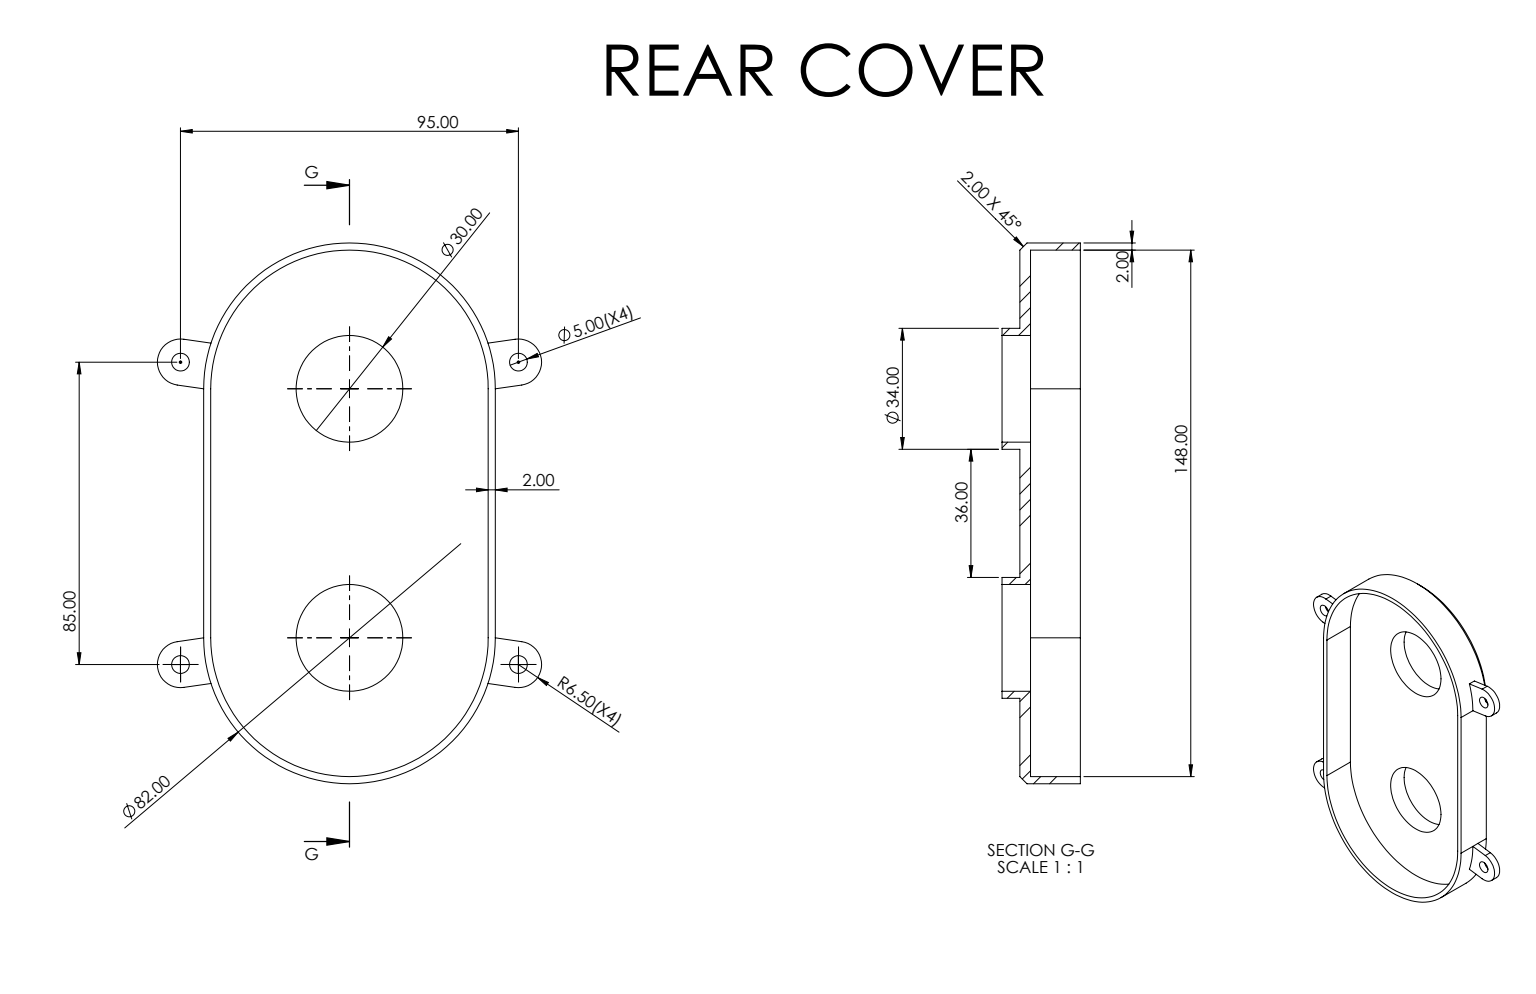
ISO-10303-21;
HEADER;
FILE_DESCRIPTION (('STEP AP214'),
    '1' );
FILE_NAME ('REAR COVER.step',
    '2026-10-24T00:51:42',
    ( '' ),
    ( '' ),
    'SwSTEP 2.0',
    'SolidWorks 2025',
    '' );
FILE_SCHEMA (( 'AUTOMOTIVE_DESIGN' ));
ENDSEC;

DATA;
#19=DIRECTION ( 'NONE',  ( -0.000000000000000000, -1.000000000000000000, -0.000000000000000000 ) ) ;
#57=VERTEX_POINT ( 'NONE', #20717 ) ;
#64=DIRECTION ( 'NONE',  ( 0.000000000000000000, 1.000000000000000000, 0.000000000000000000 ) ) ;
#78=CARTESIAN_POINT ( 'NONE',  ( 35.00000000000000000, 13.99999999999999822, 15.00000000000002132 ) ) ;
#92=EDGE_LOOP ( 'NONE', ( #21814, #17225, #4726, #11812 ) ) ;
#97=EDGE_CURVE ( 'NONE', #13097, #7488, #538, .T. ) ;
#135=EDGE_LOOP ( 'NONE', ( #20964, #9442, #3465, #7281 ) ) ;
#137=CARTESIAN_POINT ( 'NONE',  ( 42.50000000000000000, 10.00000000000000000, 47.49999999999999289 ) ) ;
#138=DIRECTION ( 'NONE',  ( -0.000000000000000000, -1.000000000000000000, -0.000000000000000000 ) ) ;
#146=VECTOR ( 'NONE', #10611, 1000.000000000000000 ) ;
#147=CARTESIAN_POINT ( 'NONE',  ( 42.50000000000000000, 7.000000000000000000, 47.49999999999999289 ) ) ;
#169=AXIS2_PLACEMENT_3D ( 'NONE', #17860, #14739, #16123 ) ;
#179=AXIS2_PLACEMENT_3D ( 'NONE', #12084, #11739, #22064 ) ;
#183=CARTESIAN_POINT ( 'NONE',  ( -42.49999999999996447, 7.000000000000000000, -47.50000000000000711 ) ) ;
#184=CYLINDRICAL_SURFACE ( 'NONE', #1331, 6.499999999999999112 ) ;
#185=AXIS2_PLACEMENT_3D ( 'NONE', #17657, #15929, #17553 ) ;
#197=LINE ( 'NONE', #10969, #5945 ) ;
#198=DIRECTION ( 'NONE',  ( -0.1421319796954322312, 0.000000000000000000, -0.9898477157360405787 ) ) ;
#202=CARTESIAN_POINT ( 'NONE',  ( -35.00000000000000000, 14.00000000000000000, 39.00000000000002132 ) ) ;
#242=EDGE_LOOP ( 'NONE', ( #11934, #16526 ) ) ;
#246=ORIENTED_EDGE ( 'NONE', *, *, #18367, .T. ) ;
#255=CARTESIAN_POINT ( 'NONE',  ( 35.00000000000000000, 17.00000000000000000, -40.99999999999997868 ) ) ;
#267=EDGE_LOOP ( 'NONE', ( #12609, #14006, #18826, #6601, #2906, #9922, #5735, #20678 ) ) ;
#279=ORIENTED_EDGE ( 'NONE', *, *, #15136, .F. ) ;
#287=AXIS2_PLACEMENT_3D ( 'NONE', #18901, #20854, #8577 ) ;
#292=DIRECTION ( 'NONE',  ( 0.000000000000000000, -1.000000000000000000, 0.000000000000000000 ) ) ;
#328=CARTESIAN_POINT ( 'NONE',  ( -35.00000000000000000, 17.00000000000000000, 2.365113165210053967E-14 ) ) ;
#336=VECTOR ( 'NONE', #1062, 1000.000000000000000 ) ;
#359=EDGE_CURVE ( 'NONE', #22631, #14416, #10776, .T. ) ;
#360=ORIENTED_EDGE ( 'NONE', *, *, #18003, .F. ) ;
#362=CARTESIAN_POINT ( 'NONE',  ( 35.00000000000000000, 0.000000000000000000, 2.365113165210053967E-14 ) ) ;
#398=EDGE_LOOP ( 'NONE', ( #11515, #3826 ) ) ;
#405=CARTESIAN_POINT ( 'NONE',  ( -41.39271818392636959, 10.00000000000000000, -5.943569790512535533 ) ) ;
#416=CYLINDRICAL_SURFACE ( 'NONE', #20007, 2.500000000000002220 ) ;
#419=ORIENTED_EDGE ( 'NONE', *, *, #14863, .F. ) ;
#424=DIRECTION ( 'NONE',  ( 0.000000000000000000, -1.000000000000000000, 0.000000000000000000 ) ) ;
#428=DIRECTION ( 'NONE',  ( 0.000000000000000000, 0.000000000000000000, -1.000000000000000000 ) ) ;
#452=DIRECTION ( 'NONE',  ( -0.000000000000000000, -1.000000000000000000, -0.000000000000000000 ) ) ;
#468=DIRECTION ( 'NONE',  ( 0.000000000000000000, 1.000000000000000000, 0.000000000000000000 ) ) ;
#472=ORIENTED_EDGE ( 'NONE', *, *, #15222, .T. ) ;
#482=ORIENTED_EDGE ( 'NONE', *, *, #4999, .F. ) ;
#484=DIRECTION ( 'NONE',  ( -0.9898477157360406897, 0.000000000000000000, -0.1421319796954317316 ) ) ;
#493=CARTESIAN_POINT ( 'NONE',  ( 47.83731665821558465, 6.999999999999999112, 38.93845529828710283 ) ) ;
#510=DIRECTION ( 'NONE',  ( 0.000000000000000000, 0.000000000000000000, 1.000000000000000000 ) ) ;
#538=CIRCLE ( 'NONE', #12595, 15.00000000000000000 ) ;
#552=FACE_BOUND ( 'NONE', #22629, .T. ) ;
#565=ADVANCED_FACE ( 'NONE', ( #8537 ), #7046, .F. ) ;
#574=CARTESIAN_POINT ( 'NONE',  ( 35.00000000000000000, 22.00000000000000355, 17.00000000000002487 ) ) ;
#594=EDGE_CURVE ( 'NONE', #9609, #19656, #19896, .T. ) ;
#608=AXIS2_PLACEMENT_3D ( 'NONE', #8171, #20770, #9889 ) ;
#628=ORIENTED_EDGE ( 'NONE', *, *, #16506, .F. ) ;
#630=DIRECTION ( 'NONE',  ( 0.000000000000000000, -1.000000000000000000, 0.000000000000000000 ) ) ;
#639=CARTESIAN_POINT ( 'NONE',  ( 42.50000000000000000, 7.000000000000000000, 49.99999999999999289 ) ) ;
#661=FACE_OUTER_BOUND ( 'NONE', #1127, .T. ) ;
#668=VERTEX_POINT ( 'NONE', #2002 ) ;
#693=CARTESIAN_POINT ( 'NONE',  ( 35.00000000000000000, 15.00000000000000000, -40.99999999999997868 ) ) ;
#716=CIRCLE ( 'NONE', #14971, 15.00000000000000000 ) ;
#718=SHAPE_REPRESENTATION_RELATIONSHIP ( 'NONE' , 'NONE' ,  #15726, #21138 ) ;
#727=FACE_OUTER_BOUND ( 'NONE', #1242, .T. ) ;
#748=EDGE_CURVE ( 'NONE', #17126, #21624, #7387, .T. ) ;
#751=FACE_OUTER_BOUND ( 'NONE', #92, .T. ) ;
#752=CARTESIAN_POINT ( 'NONE',  ( -35.00000000000000000, 17.00000000000000000, 41.00000000000002132 ) ) ;
#807=ADVANCED_FACE ( 'NONE', ( #13643, #2280 ), #20659, .T. ) ;
#809=EDGE_LOOP ( 'NONE', ( #12173, #12291, #2991, #3318 ) ) ;
#816=LINE ( 'NONE', #2658, #1235 ) ;
#837=CARTESIAN_POINT ( 'NONE',  ( -42.49999999999996447, 10.00000000000000000, -54.00000000000000711 ) ) ;
#855=ADVANCED_FACE ( 'NONE', ( #10324, #6796 ), #5093, .F. ) ;
#865=DIRECTION ( 'NONE',  ( -0.000000000000000000, 1.000000000000000000, -0.000000000000000000 ) ) ;
#883=CARTESIAN_POINT ( 'NONE',  ( -35.00000000000000000, 17.00000000000000000, -40.99999999999997868 ) ) ;
#886=FACE_OUTER_BOUND ( 'NONE', #3171, .T. ) ;
#940=DIRECTION ( 'NONE',  ( 0.000000000000000000, 0.000000000000000000, -1.000000000000000000 ) ) ;
#948=DIRECTION ( 'NONE',  ( 0.000000000000000000, 0.000000000000000000, -1.000000000000000000 ) ) ;
#963=CIRCLE ( 'NONE', #18169, 2.500000000000002220 ) ;
#968=VERTEX_POINT ( 'NONE', #6113 ) ;
#972=ORIENTED_EDGE ( 'NONE', *, *, #12220, .F. ) ;
#984=DIRECTION ( 'NONE',  ( 0.000000000000000000, 0.000000000000000000, -1.000000000000000000 ) ) ;
#1006=CIRCLE ( 'NONE', #13433, 39.00000000000000000 ) ;
#1009=CARTESIAN_POINT ( 'NONE',  ( 42.49999999999998579, 7.000000000000000000, -49.99999999999997868 ) ) ;
#1013=ORIENTED_EDGE ( 'NONE', *, *, #6207, .T. ) ;
#1017=DIRECTION ( 'NONE',  ( -0.000000000000000000, 1.000000000000000000, -0.000000000000000000 ) ) ;
#1032=CARTESIAN_POINT ( 'NONE',  ( 35.00000000000000000, 0.000000000000000000, -40.99999999999997868 ) ) ;
#1038=DIRECTION ( 'NONE',  ( 0.000000000000000000, 0.000000000000000000, -1.000000000000000000 ) ) ;
#1054=VERTEX_POINT ( 'NONE', #20767 ) ;
#1062=DIRECTION ( 'NONE',  ( -0.000000000000000000, -1.000000000000000000, -0.000000000000000000 ) ) ;
#1091=CARTESIAN_POINT ( 'NONE',  ( -28.52469787935782364, 7.000000000000000000, 4.095854054471899985 ) ) ;
#1096=DIRECTION ( 'NONE',  ( 0.000000000000000000, 0.000000000000000000, -1.000000000000000000 ) ) ;
#1120=FACE_OUTER_BOUND ( 'NONE', #7332, .T. ) ;
#1127=EDGE_LOOP ( 'NONE', ( #10984, #4974, #21316, #12105 ) ) ;
#1167=LINE ( 'NONE', #8160, #14153 ) ;
#1191=DIRECTION ( 'NONE',  ( -0.1421319796954317316, 0.000000000000000000, -0.9898477157360405787 ) ) ;
#1221=CARTESIAN_POINT ( 'NONE',  ( 41.39271818392636959, 7.000000000000000000, -5.943569790512535533 ) ) ;
#1235=VECTOR ( 'NONE', #4378, 1000.000000000000000 ) ;
#1242=EDGE_LOOP ( 'NONE', ( #6996, #21007, #22630, #22192 ) ) ;
#1265=ORIENTED_EDGE ( 'NONE', *, *, #20237, .T. ) ;
#1278=CARTESIAN_POINT ( 'NONE',  ( -35.00000000000000000, 17.00000000000000000, 41.00000000000002132 ) ) ;
#1283=VECTOR ( 'NONE', #11816, 1000.000000000000000 ) ;
#1317=DIRECTION ( 'NONE',  ( -1.000000000000000000, 0.000000000000000000, 0.000000000000000000 ) ) ;
#1331=AXIS2_PLACEMENT_3D ( 'NONE', #5809, #12782, #5471 ) ;
#1359=FACE_OUTER_BOUND ( 'NONE', #5225, .T. ) ;
#1386=CIRCLE ( 'NONE', #14175, 17.00000000000000000 ) ;
#1411=FACE_OUTER_BOUND ( 'NONE', #8286, .T. ) ;
#1430=ORIENTED_EDGE ( 'NONE', *, *, #18003, .T. ) ;
#1432=CARTESIAN_POINT ( 'NONE',  ( 35.00000000000000000, 14.00000000000000000, -38.99999999999997868 ) ) ;
#1457=ORIENTED_EDGE ( 'NONE', *, *, #7090, .T. ) ;
#1460=CARTESIAN_POINT ( 'NONE',  ( -28.52469787935786982, 10.00000000000000000, -4.095854054471906203 ) ) ;
#1464=ORIENTED_EDGE ( 'NONE', *, *, #5972, .F. ) ;
#1470=LINE ( 'NONE', #13928, #19264 ) ;
#1486=ORIENTED_EDGE ( 'NONE', *, *, #22195, .T. ) ;
#1488=( NAMED_UNIT ( * ) PLANE_ANGLE_UNIT ( ) SI_UNIT ( $, .RADIAN. ) );
#1495=DIRECTION ( 'NONE',  ( 0.000000000000000000, 0.000000000000000000, -1.000000000000000000 ) ) ;
#1522=EDGE_LOOP ( 'NONE', ( #3610, #7248, #14036, #10775 ) ) ;
#1530=ORIENTED_EDGE ( 'NONE', *, *, #20547, .F. ) ;
#1558=DIRECTION ( 'NONE',  ( 0.9898477157360406897, 0.000000000000000000, -0.1421319796954317316 ) ) ;
#1565=DIRECTION ( 'NONE',  ( 0.000000000000000000, -1.000000000000000000, 0.000000000000000000 ) ) ;
#1567=DIRECTION ( 'NONE',  ( -0.1421319796954317316, 0.000000000000000000, 0.9898477157360405787 ) ) ;
#1575=CARTESIAN_POINT ( 'NONE',  ( -35.00000000000000000, 17.00000000000000000, 2.365113165210053967E-14 ) ) ;
#1579=VECTOR ( 'NONE', #452, 1000.000000000000000 ) ;
#1582=ORIENTED_EDGE ( 'NONE', *, *, #6936, .F. ) ;
#1607=ADVANCED_FACE ( 'NONE', ( #10937 ), #2474, .F. ) ;
#1632=ADVANCED_FACE ( 'NONE', ( #751 ), #21373, .F. ) ;
#1641=CARTESIAN_POINT ( 'NONE',  ( 0.000000000000000000, 7.000000000000000000, 0.000000000000000000 ) ) ;
#1648=CARTESIAN_POINT ( 'NONE',  ( 0.000000000000000000, 0.000000000000000000, 0.000000000000000000 ) ) ;
#1691=VERTEX_POINT ( 'NONE', #17698 ) ;
#1693=CIRCLE ( 'NONE', #13357, 41.00000000000000000 ) ;
#1698=DIRECTION ( 'NONE',  ( 0.000000000000000000, 0.000000000000000000, -1.000000000000000000 ) ) ;
#1727=PRODUCT_CONTEXT ( 'NONE', #18977, 'mechanical' ) ;
#1744=LINE ( 'NONE', #12270, #4214 ) ;
#1755=DIRECTION ( 'NONE',  ( 0.1421319796954317316, 0.000000000000000000, 0.9898477157360405787 ) ) ;
#1810=EDGE_CURVE ( 'NONE', #10947, #5838, #8753, .T. ) ;
#1814=DIRECTION ( 'NONE',  ( 0.000000000000000000, -0.000000000000000000, 1.000000000000000000 ) ) ;
#1821=CARTESIAN_POINT ( 'NONE',  ( 42.49999999999998579, 10.00000000000000000, -53.99999999999997868 ) ) ;
#1844=CARTESIAN_POINT ( 'NONE',  ( -35.00000000000000000, -15.00000000000000000, 15.00000000000002132 ) ) ;
#1861=CYLINDRICAL_SURFACE ( 'NONE', #185, 17.00000000000000000 ) ;
#1869=VERTEX_POINT ( 'NONE', #4975 ) ;
#1882=ORIENTED_EDGE ( 'NONE', *, *, #8202, .F. ) ;
#1921=VECTOR ( 'NONE', #2869, 1000.000000000000000 ) ;
#1930=CARTESIAN_POINT ( 'NONE',  ( -35.00000000000000000, 14.00000000000000000, 2.365113165210053967E-14 ) ) ;
#1932=DIRECTION ( 'NONE',  ( 0.000000000000000000, 1.000000000000000000, 0.000000000000000000 ) ) ;
#1934=CARTESIAN_POINT ( 'NONE',  ( 41.39271818392636959, 10.00000000000000000, -5.943569790512535533 ) ) ;
#1937=AXIS2_PLACEMENT_3D ( 'NONE', #10361, #1558, #17361 ) ;
#1949=CARTESIAN_POINT ( 'NONE',  ( 35.00000000000000000, -15.00000000000000000, 2.255140518769849223E-14 ) ) ;
#1979=DIRECTION ( 'NONE',  ( 0.000000000000000000, 0.000000000000000000, 1.000000000000000000 ) ) ;
#1986=LINE ( 'NONE', #16071, #20757 ) ;
#1989=VECTOR ( 'NONE', #13933, 1000.000000000000000 ) ;
#2002=CARTESIAN_POINT ( 'NONE',  ( 36.06598984771572702, 7.000000000000000000, -48.42385786802028491 ) ) ;
#2042=DIRECTION ( 'NONE',  ( 0.000000000000000000, -0.000000000000000000, -1.000000000000000000 ) ) ;
#2066=DIRECTION ( 'NONE',  ( 1.000000000000000000, 0.000000000000000000, 0.000000000000000000 ) ) ;
#2069=CARTESIAN_POINT ( 'NONE',  ( -47.83731665821558465, 10.00000000000000000, 38.93845529828710283 ) ) ;
#2070=ADVANCED_FACE ( 'NONE', ( #4157, #11129 ), #5758, .T. ) ;
#2076=CARTESIAN_POINT ( 'NONE',  ( 42.50000000000000000, 10.00000000000000000, 44.99999999999999289 ) ) ;
#2124=DIRECTION ( 'NONE',  ( -0.1421319796954322312, 0.000000000000000000, 0.9898477157360405787 ) ) ;
#2151=ORIENTED_EDGE ( 'NONE', *, *, #14754, .T. ) ;
#2156=CARTESIAN_POINT ( 'NONE',  ( -35.00000000000000000, 0.000000000000000000, -40.99999999999997868 ) ) ;
#2157=CARTESIAN_POINT ( 'NONE',  ( 0.000000000000000000, 10.00000000000000000, 0.000000000000000000 ) ) ;
#2214=FACE_OUTER_BOUND ( 'NONE', #13033, .T. ) ;
#2237=CARTESIAN_POINT ( 'NONE',  ( -35.00000000000000000, 13.99999999999999822, 2.255140518769849223E-14 ) ) ;
#2242=CARTESIAN_POINT ( 'NONE',  ( 42.49999999999998579, 10.00000000000000000, -53.99999999999997868 ) ) ;
#2247=CARTESIAN_POINT ( 'NONE',  ( -42.49999999999996447, 10.00000000000000000, -47.50000000000000711 ) ) ;
#2268=DIRECTION ( 'NONE',  ( 0.000000000000000000, -1.000000000000000000, 0.000000000000000000 ) ) ;
#2271=CARTESIAN_POINT ( 'NONE',  ( 42.50000000000000000, 7.000000000000000000, 47.49999999999999289 ) ) ;
#2272=DIRECTION ( 'NONE',  ( 0.000000000000000000, 0.000000000000000000, 1.000000000000000000 ) ) ;
#2280=FACE_BOUND ( 'NONE', #20023, .T. ) ;
#2309=VECTOR ( 'NONE', #22199, 1000.000000000000000 ) ;
#2314=CIRCLE ( 'NONE', #18793, 39.00000000000001421 ) ;
#2320=ORIENTED_EDGE ( 'NONE', *, *, #16902, .T. ) ;
#2333=DIRECTION ( 'NONE',  ( -0.000000000000000000, 1.000000000000000000, -0.000000000000000000 ) ) ;
#2334=CARTESIAN_POINT ( 'NONE',  ( -35.00000000000000000, -15.00000000000000000, 2.255140518769849223E-14 ) ) ;
#2351=CARTESIAN_POINT ( 'NONE',  ( 41.39271818392635538, 10.00000000000000000, 5.943569790512533757 ) ) ;
#2360=ORIENTED_EDGE ( 'NONE', *, *, #12885, .T. ) ;
#2367=VECTOR ( 'NONE', #10808, 1000.000000000000000 ) ;
#2431=AXIS2_PLACEMENT_3D ( 'NONE', #11425, #7878, #7759 ) ;
#2470=EDGE_CURVE ( 'NONE', #5472, #3556, #22295, .T. ) ;
#2471=EDGE_LOOP ( 'NONE', ( #2738, #11209 ) ) ;
#2474=CYLINDRICAL_SURFACE ( 'NONE', #16918, 15.00000000000000000 ) ;
#2482=VECTOR ( 'NONE', #1567, 1000.000000000000114 ) ;
#2485=AXIS2_PLACEMENT_3D ( 'NONE', #6864, #20850, #13709 ) ;
#2513=CARTESIAN_POINT ( 'NONE',  ( -35.00000000000000000, 22.00000000000000711, 2.255140518769849223E-14 ) ) ;
#2520=LINE ( 'NONE', #4463, #14838 ) ;
#2557=DIRECTION ( 'NONE',  ( 0.000000000000000000, -1.000000000000000000, 0.000000000000000000 ) ) ;
#2637=EDGE_CURVE ( 'NONE', #16920, #5292, #18981, .T. ) ;
#2651=DIRECTION ( 'NONE',  ( 0.000000000000000000, -1.000000000000000000, 0.000000000000000000 ) ) ;
#2653=EDGE_CURVE ( 'NONE', #14416, #22631, #5060, .T. ) ;
#2658=CARTESIAN_POINT ( 'NONE',  ( -36.06598984771573413, 10.00000000000000000, 48.42385786802029912 ) ) ;
#2734=CARTESIAN_POINT ( 'NONE',  ( 35.00000000000000000, 13.99999999999999822, -14.99999999999997691 ) ) ;
#2737=DIRECTION ( 'NONE',  ( 0.000000000000000000, 1.000000000000000000, 0.000000000000000000 ) ) ;
#2738=ORIENTED_EDGE ( 'NONE', *, *, #7323, .F. ) ;
#2767=ORIENTED_EDGE ( 'NONE', *, *, #22107, .F. ) ;
#2795=DIRECTION ( 'NONE',  ( -0.000000000000000000, 1.000000000000000000, -0.000000000000000000 ) ) ;
#2798=VECTOR ( 'NONE', #7146, 1000.000000000000000 ) ;
#2800=PRODUCT_DEFINITION_CONTEXT ( 'detailed design', #13389, 'design' ) ;
#2815=ORIENTED_EDGE ( 'NONE', *, *, #3808, .F. ) ;
#2833=LINE ( 'NONE', #13339, #2309 ) ;
#2869=DIRECTION ( 'NONE',  ( -0.000000000000000000, -1.000000000000000000, -0.000000000000000000 ) ) ;
#2879=ADVANCED_FACE ( 'NONE', ( #22518 ), #19072, .F. ) ;
#2888=VECTOR ( 'NONE', #11317, 1000.000000000000000 ) ;
#2890=AXIS2_PLACEMENT_3D ( 'NONE', #7003, #6777, #13959 ) ;
#2892=EDGE_LOOP ( 'NONE', ( #1882, #5395 ) ) ;
#2899=EDGE_CURVE ( 'NONE', #1869, #7355, #7256, .T. ) ;
#2906=ORIENTED_EDGE ( 'NONE', *, *, #3732, .T. ) ;
#2956=PLANE ( 'NONE',  #21445 ) ;
#2991=ORIENTED_EDGE ( 'NONE', *, *, #3871, .T. ) ;
#3007=ORIENTED_EDGE ( 'NONE', *, *, #12807, .F. ) ;
#3018=ORIENTED_EDGE ( 'NONE', *, *, #5005, .F. ) ;
#3027=EDGE_LOOP ( 'NONE', ( #19847, #19122, #3846, #7657 ) ) ;
#3041=FACE_BOUND ( 'NONE', #7156, .T. ) ;
#3052=ORIENTED_EDGE ( 'NONE', *, *, #5972, .T. ) ;
#3065=CARTESIAN_POINT ( 'NONE',  ( -42.50000000000000000, 10.00000000000000000, 47.49999999999999289 ) ) ;
#3069=CARTESIAN_POINT ( 'NONE',  ( -42.50000000000000000, 10.00000000000000000, 47.49999999999999289 ) ) ;
#3072=AXIS2_PLACEMENT_3D ( 'NONE', #4866, #20225, #18842 ) ;
#3079=FACE_OUTER_BOUND ( 'NONE', #16197, .T. ) ;
#3083=ORIENTED_EDGE ( 'NONE', *, *, #12925, .F. ) ;
#3092=EDGE_LOOP ( 'NONE', ( #20794, #13463 ) ) ;
#3117=ORIENTED_EDGE ( 'NONE', *, *, #14660, .F. ) ;
#3130=DIRECTION ( 'NONE',  ( 0.9898477157360406897, 0.000000000000000000, 0.1421319796954317316 ) ) ;
#3134=EDGE_CURVE ( 'NONE', #9062, #12985, #18351, .T. ) ;
#3151=VERTEX_POINT ( 'NONE', #22144 ) ;
#3162=EDGE_CURVE ( 'NONE', #6209, #12263, #7939, .T. ) ;
#3168=VECTOR ( 'NONE', #14054, 999.9999999999998863 ) ;
#3171=EDGE_LOOP ( 'NONE', ( #3117, #19504, #7395, #8158 ) ) ;
#3185=DIRECTION ( 'NONE',  ( 0.000000000000000000, 1.000000000000000000, 0.000000000000000000 ) ) ;
#3196=EDGE_LOOP ( 'NONE', ( #19684, #11491, #11820, #18594 ) ) ;
#3240=EDGE_CURVE ( 'NONE', #5472, #968, #3575, .T. ) ;
#3258=EDGE_LOOP ( 'NONE', ( #279, #7361, #12926, #9656 ) ) ;
#3270=LINE ( 'NONE', #12405, #4800 ) ;
#3305=FACE_OUTER_BOUND ( 'NONE', #5612, .T. ) ;
#3310=PLANE ( 'NONE',  #8420 ) ;
#3318=ORIENTED_EDGE ( 'NONE', *, *, #5798, .T. ) ;
#3325=EDGE_LOOP ( 'NONE', ( #14607, #3483, #8538, #18494, #14886 ) ) ;
#3380=CARTESIAN_POINT ( 'NONE',  ( 42.49999999999998579, 10.00000000000000000, -47.49999999999997868 ) ) ;
#3382=ORIENTED_EDGE ( 'NONE', *, *, #8745, .F. ) ;
#3420=ORIENTED_EDGE ( 'NONE', *, *, #22107, .T. ) ;
#3455=CIRCLE ( 'NONE', #8931, 41.00000000000000000 ) ;
#3465=ORIENTED_EDGE ( 'NONE', *, *, #4547, .T. ) ;
#3482=ADVANCED_FACE ( 'NONE', ( #10754 ), #19600, .T. ) ;
#3483=ORIENTED_EDGE ( 'NONE', *, *, #3782, .F. ) ;
#3492=EDGE_CURVE ( 'NONE', #8659, #11088, #9060, .T. ) ;
#3507=CARTESIAN_POINT ( 'NONE',  ( 42.49999999999998579, 10.00000000000000000, -44.99999999999997868 ) ) ;
#3509=DIRECTION ( 'NONE',  ( 0.000000000000000000, 0.000000000000000000, -1.000000000000000000 ) ) ;
#3529=CARTESIAN_POINT ( 'NONE',  ( -42.50000000000000000, 10.00000000000000000, 47.49999999999999289 ) ) ;
#3535=CIRCLE ( 'NONE', #6816, 17.00000000000000000 ) ;
#3551=CYLINDRICAL_SURFACE ( 'NONE', #287, 6.499999999999999112 ) ;
#3554=DIRECTION ( 'NONE',  ( 0.1421319796954317316, 0.000000000000000000, -0.9898477157360405787 ) ) ;
#3556=VERTEX_POINT ( 'NONE', #574 ) ;
#3575=LINE ( 'NONE', #8602, #7278 ) ;
#3598=VECTOR ( 'NONE', #7421, 1000.000000000000000 ) ;
#3610=ORIENTED_EDGE ( 'NONE', *, *, #97, .T. ) ;
#3623=EDGE_CURVE ( 'NONE', #22687, #9796, #7787, .T. ) ;
#3625=FACE_BOUND ( 'NONE', #8762, .T. ) ;
#3626=DIRECTION ( 'NONE',  ( 0.000000000000000000, -1.000000000000000000, 0.000000000000000000 ) ) ;
#3632=ORIENTED_EDGE ( 'NONE', *, *, #16597, .F. ) ;
#3633=ORIENTED_EDGE ( 'NONE', *, *, #2637, .T. ) ;
#3653=CARTESIAN_POINT ( 'NONE',  ( -42.49999999999996447, 10.00000000000000000, -50.00000000000000711 ) ) ;
#3654=DIRECTION ( 'NONE',  ( 0.000000000000000000, 0.000000000000000000, -1.000000000000000000 ) ) ;
#3666=CARTESIAN_POINT ( 'NONE',  ( 35.00000000000000000, 17.00000000000000000, -38.99999999999999289 ) ) ;
#3694=CARTESIAN_POINT ( 'NONE',  ( -41.39271818392631985, 7.000000000000000000, 5.943569790512528428 ) ) ;
#3701=ORIENTED_EDGE ( 'NONE', *, *, #14762, .T. ) ;
#3723=DIRECTION ( 'NONE',  ( 0.000000000000000000, 0.000000000000000000, -1.000000000000000000 ) ) ;
#3732=EDGE_CURVE ( 'NONE', #8574, #9457, #11569, .T. ) ;
#3744=LINE ( 'NONE', #9429, #22652 ) ;
#3754=CARTESIAN_POINT ( 'NONE',  ( -42.49999999999996447, 7.000000000000000000, -47.50000000000000711 ) ) ;
#3772=ORIENTED_EDGE ( 'NONE', *, *, #9384, .T. ) ;
#3782=EDGE_CURVE ( 'NONE', #9695, #9796, #15672, .T. ) ;
#3797=CIRCLE ( 'NONE', #16596, 2.500000000000002220 ) ;
#3808=EDGE_CURVE ( 'NONE', #8847, #16743, #12022, .T. ) ;
#3812=MECHANICAL_DESIGN_GEOMETRIC_PRESENTATION_REPRESENTATION('',(#13668),#11862);
#3826=ORIENTED_EDGE ( 'NONE', *, *, #4433, .F. ) ;
#3832=EDGE_LOOP ( 'NONE', ( #10837, #10650, #12585, #7543 ) ) ;
#3833=CARTESIAN_POINT ( 'NONE',  ( 35.00000000000000000, 0.000000000000000000, 2.365113165210053967E-14 ) ) ;
#3846=ORIENTED_EDGE ( 'NONE', *, *, #3162, .T. ) ;
#3858=LINE ( 'NONE', #11145, #15632 ) ;
#3871=EDGE_CURVE ( 'NONE', #1691, #6084, #197, .T. ) ;
#3877=AXIS2_PLACEMENT_3D ( 'NONE', #5239, #3185, #19221 ) ;
#3904=AXIS2_PLACEMENT_3D ( 'NONE', #2334, #21939, #12752 ) ;
#3908=CYLINDRICAL_SURFACE ( 'NONE', #3989, 15.00000000000000000 ) ;
#3909=VERTEX_POINT ( 'NONE', #7192 ) ;
#3938=ORIENTED_EDGE ( 'NONE', *, *, #15815, .F. ) ;
#3948=VECTOR ( 'NONE', #21942, 1000.000000000000000 ) ;
#3967=VERTEX_POINT ( 'NONE', #19463 ) ;
#3985=CIRCLE ( 'NONE', #5431, 41.00000000000000000 ) ;
#3989=AXIS2_PLACEMENT_3D ( 'NONE', #1949, #7334, #5502 ) ;
#3991=VERTEX_POINT ( 'NONE', #13233 ) ;
#4001=PLANE ( 'NONE',  #6171 ) ;
#4010=ADVANCED_FACE ( 'NONE', ( #661 ), #13131, .F. ) ;
#4031=FACE_OUTER_BOUND ( 'NONE', #1522, .T. ) ;
#4051=ORIENTED_EDGE ( 'NONE', *, *, #20533, .F. ) ;
#4074=VECTOR ( 'NONE', #2557, 1000.000000000000000 ) ;
#4101=CARTESIAN_POINT ( 'NONE',  ( -35.00000000000000000, 25.00000000000000000, 2.365113165210053967E-14 ) ) ;
#4114=DIRECTION ( 'NONE',  ( 0.000000000000000000, 0.000000000000000000, -1.000000000000000000 ) ) ;
#4116=FACE_OUTER_BOUND ( 'NONE', #19797, .T. ) ;
#4157=FACE_BOUND ( 'NONE', #9390, .T. ) ;
#4173=FACE_OUTER_BOUND ( 'NONE', #135, .T. ) ;
#4176=CARTESIAN_POINT ( 'NONE',  ( -35.00000000000000000, 10.00000000000000000, -40.99999999999997868 ) ) ;
#4180=CIRCLE ( 'NONE', #10015, 17.00000000000000000 ) ;
#4196=DIRECTION ( 'NONE',  ( 0.9898477157360405787, 0.000000000000000000, 0.1421319796954322312 ) ) ;
#4214=VECTOR ( 'NONE', #19, 1000.000000000000000 ) ;
#4228=DIRECTION ( 'NONE',  ( -0.000000000000000000, -1.000000000000000000, -0.000000000000000000 ) ) ;
#4246=CARTESIAN_POINT ( 'NONE',  ( 48.93401015228424455, 10.00000000000000000, -46.57614213197967956 ) ) ;
#4273=EDGE_CURVE ( 'NONE', #10917, #1054, #3858, .T. ) ;
#4280=CARTESIAN_POINT ( 'NONE',  ( -41.39271818392636959, 10.00000000000000000, -5.943569790512535533 ) ) ;
#4289=CARTESIAN_POINT ( 'NONE',  ( -35.00000000000000000, 15.00000000000000000, 2.365113165210053967E-14 ) ) ;
#4293=CIRCLE ( 'NONE', #4608, 6.499999999999999112 ) ;
#4294=ORIENTED_EDGE ( 'NONE', *, *, #6266, .F. ) ;
#4295=CYLINDRICAL_SURFACE ( 'NONE', #11531, 2.500000000000002220 ) ;
#4300=VECTOR ( 'NONE', #18816, 1000.000000000000000 ) ;
#4320=FACE_OUTER_BOUND ( 'NONE', #18037, .T. ) ;
#4355=LINE ( 'NONE', #9843, #5362 ) ;
#4356=EDGE_CURVE ( 'NONE', #8405, #10917, #16739, .T. ) ;
#4359=ORIENTED_EDGE ( 'NONE', *, *, #9254, .F. ) ;
#4378=DIRECTION ( 'NONE',  ( 0.000000000000000000, -1.000000000000000000, 0.000000000000000000 ) ) ;
#4381=VERTEX_POINT ( 'NONE', #9191 ) ;
#4406=ORIENTED_EDGE ( 'NONE', *, *, #9942, .T. ) ;
#4409=DIRECTION ( 'NONE',  ( 0.000000000000000000, 0.000000000000000000, -1.000000000000000000 ) ) ;
#4418=ORIENTED_EDGE ( 'NONE', *, *, #3492, .T. ) ;
#4426=EDGE_CURVE ( 'NONE', #8747, #14227, #18943, .T. ) ;
#4433=EDGE_CURVE ( 'NONE', #11772, #6084, #7969, .T. ) ;
#4438=ORIENTED_EDGE ( 'NONE', *, *, #17655, .F. ) ;
#4453=VECTOR ( 'NONE', #10143, 1000.000000000000114 ) ;
#4463=CARTESIAN_POINT ( 'NONE',  ( -35.00000000000000000, 0.000000000000000000, -40.99999999999997868 ) ) ;
#4491=( LENGTH_UNIT ( ) NAMED_UNIT ( * ) SI_UNIT ( .MILLI., .METRE. ) );
#4495=VECTOR ( 'NONE', #8025, 1000.000000000000000 ) ;
#4510=ORIENTED_EDGE ( 'NONE', *, *, #22195, .F. ) ;
#4526=ORIENTED_EDGE ( 'NONE', *, *, #2470, .F. ) ;
#4529=ORIENTED_EDGE ( 'NONE', *, *, #9755, .F. ) ;
#4547=EDGE_CURVE ( 'NONE', #13043, #9609, #8486, .T. ) ;
#4554=ORIENTED_EDGE ( 'NONE', *, *, #5776, .T. ) ;
#4582=CYLINDRICAL_SURFACE ( 'NONE', #4905, 41.00000000000000000 ) ;
#4598=DIRECTION ( 'NONE',  ( -0.000000000000000000, 1.000000000000000000, -0.000000000000000000 ) ) ;
#4604=AXIS2_PLACEMENT_3D ( 'NONE', #11825, #4963, #18944 ) ;
#4608=AXIS2_PLACEMENT_3D ( 'NONE', #147, #7142, #7375 ) ;
#4630=CARTESIAN_POINT ( 'NONE',  ( 48.93401015228426587, 7.000000000000000000, 46.57614213197968667 ) ) ;
#4638=PLANE ( 'NONE',  #21326 ) ;
#4644=AXIS2_PLACEMENT_3D ( 'NONE', #5773, #2333, #14584 ) ;
#4650=DIRECTION ( 'NONE',  ( 0.000000000000000000, 1.000000000000000000, 0.000000000000000000 ) ) ;
#4653=PLANE ( 'NONE',  #6608 ) ;
#4675=CARTESIAN_POINT ( 'NONE',  ( -35.00000000000000000, 15.00000000000000000, -40.99999999999997868 ) ) ;
#4687=AXIS2_PLACEMENT_3D ( 'NONE', #18782, #10056, #5042 ) ;
#4695=EDGE_LOOP ( 'NONE', ( #17693, #20869, #7283, #1582 ) ) ;
#4697=DIRECTION ( 'NONE',  ( 0.000000000000000000, 0.000000000000000000, -1.000000000000000000 ) ) ;
#4711=EDGE_CURVE ( 'NONE', #8574, #668, #9822, .T. ) ;
#4716=CARTESIAN_POINT ( 'NONE',  ( 35.00000000000000000, -15.00000000000000000, 2.255140518769849223E-14 ) ) ;
#4726=ORIENTED_EDGE ( 'NONE', *, *, #13705, .F. ) ;
#4743=DIRECTION ( 'NONE',  ( 0.000000000000000000, 1.000000000000000000, 0.000000000000000000 ) ) ;
#4749=CARTESIAN_POINT ( 'NONE',  ( 42.49999999999998579, 10.00000000000000000, -49.99999999999997868 ) ) ;
#4750=CARTESIAN_POINT ( 'NONE',  ( 35.00000000000000000, 15.00000000000000000, 41.00000000000002132 ) ) ;
#4756=EDGE_LOOP ( 'NONE', ( #6381, #1486, #17696, #9217 ) ) ;
#4776=EDGE_CURVE ( 'NONE', #5656, #13337, #18797, .T. ) ;
#4800=VECTOR ( 'NONE', #19302, 999.9999999999998863 ) ;
#4837=VERTEX_POINT ( 'NONE', #2242 ) ;
#4841=ADVANCED_FACE ( 'NONE', ( #12651 ), #7514, .F. ) ;
#4843=LINE ( 'NONE', #11813, #4300 ) ;
#4846=CARTESIAN_POINT ( 'NONE',  ( -35.00000000000000000, -15.00000000000000000, -14.99999999999997691 ) ) ;
#4854=PLANE ( 'NONE',  #10166 ) ;
#4863=CARTESIAN_POINT ( 'NONE',  ( 35.00000000000000000, 7.000000000000000000, 41.00000000000002132 ) ) ;
#4866=CARTESIAN_POINT ( 'NONE',  ( 35.00000000000000000, 17.00000000000000000, 2.365113165210053967E-14 ) ) ;
#4869=CARTESIAN_POINT ( 'NONE',  ( -35.00000000000000000, 22.00000000000000355, 2.365113165210053967E-14 ) ) ;
#4897=CYLINDRICAL_SURFACE ( 'NONE', #12016, 2.500000000000002220 ) ;
#4905=AXIS2_PLACEMENT_3D ( 'NONE', #10050, #13370, #4697 ) ;
#4906=DIRECTION ( 'NONE',  ( 0.000000000000000000, 0.000000000000000000, -1.000000000000000000 ) ) ;
#4961=CARTESIAN_POINT ( 'NONE',  ( -35.00000000000000000, 0.000000000000000000, 2.365113165210053967E-14 ) ) ;
#4963=DIRECTION ( 'NONE',  ( 0.000000000000000000, -1.000000000000000000, 0.000000000000000000 ) ) ;
#4973=CARTESIAN_POINT ( 'NONE',  ( 48.93401015228424455, 10.00000000000000000, -46.57614213197967956 ) ) ;
#4974=ORIENTED_EDGE ( 'NONE', *, *, #17616, .F. ) ;
#4975=CARTESIAN_POINT ( 'NONE',  ( 35.00000000000001421, 0.000000000000000000, 39.00000000000002132 ) ) ;
#4995=DIRECTION ( 'NONE',  ( 0.000000000000000000, -0.000000000000000000, -1.000000000000000000 ) ) ;
#4999=EDGE_CURVE ( 'NONE', #12985, #6209, #9557, .T. ) ;
#5005=EDGE_CURVE ( 'NONE', #57, #13636, #3270, .T. ) ;
#5024=VERTEX_POINT ( 'NONE', #10570 ) ;
#5042=DIRECTION ( 'NONE',  ( 0.000000000000000000, 0.000000000000000000, -1.000000000000000000 ) ) ;
#5060=CIRCLE ( 'NONE', #22275, 2.500000000000002220 ) ;
#5088=AXIS2_PLACEMENT_3D ( 'NONE', #21868, #6167, #3723 ) ;
#5093=PLANE ( 'NONE',  #12578 ) ;
#5096=ORIENTED_EDGE ( 'NONE', *, *, #12555, .F. ) ;
#5129=DIRECTION ( 'NONE',  ( 0.000000000000000000, 0.000000000000000000, 1.000000000000000000 ) ) ;
#5132=FACE_OUTER_BOUND ( 'NONE', #12353, .T. ) ;
#5153=VECTOR ( 'NONE', #16231, 1000.000000000000114 ) ;
#5154=CARTESIAN_POINT ( 'NONE',  ( 35.00000000000000000, 17.00000000000000000, -38.99999999999999289 ) ) ;
#5160=PLANE ( 'NONE',  #16283 ) ;
#5166=ORIENTED_EDGE ( 'NONE', *, *, #5233, .T. ) ;
#5176=DIRECTION ( 'NONE',  ( 0.000000000000000000, 0.000000000000000000, -1.000000000000000000 ) ) ;
#5191=ORIENTED_EDGE ( 'NONE', *, *, #10332, .T. ) ;
#5223=ADVANCED_FACE ( 'NONE', ( #727 ), #5529, .T. ) ;
#5225=EDGE_LOOP ( 'NONE', ( #419, #21595, #15652, #18243 ) ) ;
#5233=EDGE_CURVE ( 'NONE', #15126, #668, #21690, .T. ) ;
#5239=CARTESIAN_POINT ( 'NONE',  ( -35.00000000000000000, 17.00000000000000000, 2.365113165210053967E-14 ) ) ;
#5245=ADVANCED_FACE ( 'NONE', ( #2214 ), #9196, .T. ) ;
#5292=VERTEX_POINT ( 'NONE', #7940 ) ;
#5312=DIRECTION ( 'NONE',  ( -1.000000000000000000, -0.000000000000000000, -0.000000000000000000 ) ) ;
#5318=CARTESIAN_POINT ( 'NONE',  ( -35.00000000000000000, 10.00000000000000000, 2.365113165210053967E-14 ) ) ;
#5323=CARTESIAN_POINT ( 'NONE',  ( -35.00000000000000000, 7.000000000000000000, 2.365113165210053967E-14 ) ) ;
#5329=DIRECTION ( 'NONE',  ( 1.000000000000000000, -0.000000000000000000, -0.000000000000000000 ) ) ;
#5354=DIRECTION ( 'NONE',  ( 0.000000000000000000, -1.000000000000000000, 0.000000000000000000 ) ) ;
#5362=VECTOR ( 'NONE', #13243, 1000.000000000000000 ) ;
#5368=FACE_OUTER_BOUND ( 'NONE', #19665, .T. ) ;
#5372=LINE ( 'NONE', #3666, #8701 ) ;
#5379=EDGE_CURVE ( 'NONE', #13337, #21700, #1167, .T. ) ;
#5395=ORIENTED_EDGE ( 'NONE', *, *, #7223, .F. ) ;
#5403=ORIENTED_EDGE ( 'NONE', *, *, #10283, .T. ) ;
#5406=PLANE ( 'NONE',  #13322 ) ;
#5410=AXIS2_PLACEMENT_3D ( 'NONE', #10783, #5636, #1979 ) ;
#5431=AXIS2_PLACEMENT_3D ( 'NONE', #5323, #8763, #15735 ) ;
#5436=CARTESIAN_POINT ( 'NONE',  ( 35.00000000000000000, 17.00000000000000000, 2.365113165210053967E-14 ) ) ;
#5471=DIRECTION ( 'NONE',  ( 0.000000000000000000, 0.000000000000000000, -1.000000000000000000 ) ) ;
#5472=VERTEX_POINT ( 'NONE', #15582 ) ;
#5502=DIRECTION ( 'NONE',  ( 0.000000000000000000, 0.000000000000000000, 1.000000000000000000 ) ) ;
#5529=CYLINDRICAL_SURFACE ( 'NONE', #9801, 6.499999999999999112 ) ;
#5536=ORIENTED_EDGE ( 'NONE', *, *, #3492, .F. ) ;
#5581=CARTESIAN_POINT ( 'NONE',  ( -35.00000000000000000, 6.999999999999999112, 41.00000000000002132 ) ) ;
#5582=DIRECTION ( 'NONE',  ( 0.000000000000000000, -1.000000000000000000, 0.000000000000000000 ) ) ;
#5596=AXIS2_PLACEMENT_3D ( 'NONE', #362, #7353, #14321 ) ;
#5597=EDGE_CURVE ( 'NONE', #22687, #4837, #14537, .T. ) ;
#5602=AXIS2_PLACEMENT_3D ( 'NONE', #405, #4196, #12990 ) ;
#5603=EDGE_LOOP ( 'NONE', ( #2360, #9910, #6653, #18837 ) ) ;
#5612=EDGE_LOOP ( 'NONE', ( #4406, #14116, #16090, #19294 ) ) ;
#5623=AXIS2_PLACEMENT_3D ( 'NONE', #12093, #12312, #10248 ) ;
#5636=DIRECTION ( 'NONE',  ( 0.000000000000000000, -1.000000000000000000, 0.000000000000000000 ) ) ;
#5643=DIRECTION ( 'NONE',  ( 0.000000000000000000, 0.000000000000000000, -1.000000000000000000 ) ) ;
#5656=VERTEX_POINT ( 'NONE', #18676 ) ;
#5666=ORIENTED_EDGE ( 'NONE', *, *, #3240, .T. ) ;
#5687=EDGE_CURVE ( 'NONE', #21104, #668, #8339, .T. ) ;
#5735=ORIENTED_EDGE ( 'NONE', *, *, #5379, .F. ) ;
#5749=CARTESIAN_POINT ( 'NONE',  ( 42.50000000000000000, 10.00000000000000000, 47.49999999999999289 ) ) ;
#5758=PLANE ( 'NONE',  #21652 ) ;
#5773=CARTESIAN_POINT ( 'NONE',  ( -42.49999999999996447, 7.000000000000000000, -47.50000000000000711 ) ) ;
#5776=EDGE_CURVE ( 'NONE', #10413, #20463, #6888, .T. ) ;
#5781=CIRCLE ( 'NONE', #21513, 6.499999999999999112 ) ;
#5798=EDGE_CURVE ( 'NONE', #6084, #11772, #6509, .T. ) ;
#5809=CARTESIAN_POINT ( 'NONE',  ( 42.50000000000000000, 10.00000000000000000, 47.49999999999999289 ) ) ;
#5820=ADVANCED_FACE ( 'NONE', ( #13939 ), #3551, .T. ) ;
#5834=DIRECTION ( 'NONE',  ( 0.000000000000000000, -1.000000000000000000, 0.000000000000000000 ) ) ;
#5838=VERTEX_POINT ( 'NONE', #13714 ) ;
#5849=VERTEX_POINT ( 'NONE', #6869 ) ;
#5877=DIRECTION ( 'NONE',  ( 0.000000000000000000, -1.000000000000000000, 0.000000000000000000 ) ) ;
#5899=ORIENTED_EDGE ( 'NONE', *, *, #17210, .T. ) ;
#5910=CARTESIAN_POINT ( 'NONE',  ( -35.00000000000000000, 7.000000000000000000, 2.365113165210053967E-14 ) ) ;
#5918=DIRECTION ( 'NONE',  ( -0.000000000000000000, 1.000000000000000000, -0.000000000000000000 ) ) ;
#5924=ADVANCED_FACE ( 'NONE', ( #12348 ), #4001, .T. ) ;
#5945=VECTOR ( 'NONE', #5582, 1000.000000000000000 ) ;
#5963=EDGE_CURVE ( 'NONE', #16920, #6360, #18189, .T. ) ;
#5972=EDGE_CURVE ( 'NONE', #3909, #16743, #21985, .T. ) ;
#5988=DIRECTION ( 'NONE',  ( 0.000000000000000000, -1.000000000000000000, 0.000000000000000000 ) ) ;
#5993=ORIENTED_EDGE ( 'NONE', *, *, #2653, .F. ) ;
#5996=DIRECTION ( 'NONE',  ( 0.000000000000000000, 0.000000000000000000, 1.000000000000000000 ) ) ;
#6003=CIRCLE ( 'NONE', #19531, 17.00000000000000000 ) ;
#6013=ORIENTED_EDGE ( 'NONE', *, *, #16529, .F. ) ;
#6016=DIRECTION ( 'NONE',  ( 0.000000000000000000, 0.000000000000000000, -1.000000000000000000 ) ) ;
#6054=DIRECTION ( 'NONE',  ( 0.000000000000000000, 0.000000000000000000, 1.000000000000000000 ) ) ;
#6057=ORIENTED_EDGE ( 'NONE', *, *, #9831, .T. ) ;
#6076=ADVANCED_FACE ( 'NONE', ( #1120 ), #18966, .F. ) ;
#6080=ORIENTED_EDGE ( 'NONE', *, *, #8804, .F. ) ;
#6084=VERTEX_POINT ( 'NONE', #11967 ) ;
#6085=CARTESIAN_POINT ( 'NONE',  ( 42.49999999999998579, 7.000000000000000000, -47.49999999999997868 ) ) ;
#6088=CARTESIAN_POINT ( 'NONE',  ( -48.93401015228422324, 7.000000000000000000, -46.57614213197970088 ) ) ;
#6093=VECTOR ( 'NONE', #9580, 1000.000000000000000 ) ;
#6107=ADVANCED_FACE ( 'NONE', ( #886 ), #7879, .T. ) ;
#6113=CARTESIAN_POINT ( 'NONE',  ( 35.00000000000000000, 17.00000000000000000, -16.99999999999997868 ) ) ;
#6123=DIRECTION ( 'NONE',  ( -0.9898477157360406897, 0.000000000000000000, 0.1421319796954317316 ) ) ;
#6156=ORIENTED_EDGE ( 'NONE', *, *, #7339, .F. ) ;
#6167=DIRECTION ( 'NONE',  ( -0.000000000000000000, -1.000000000000000000, -0.000000000000000000 ) ) ;
#6171=AXIS2_PLACEMENT_3D ( 'NONE', #14392, #16354, #198 ) ;
#6180=DIRECTION ( 'NONE',  ( -1.000000000000000000, -0.000000000000000000, -0.000000000000000000 ) ) ;
#6181=VECTOR ( 'NONE', #1565, 1000.000000000000000 ) ;
#6183=ORIENTED_EDGE ( 'NONE', *, *, #15884, .T. ) ;
#6207=EDGE_CURVE ( 'NONE', #8659, #3991, #3985, .T. ) ;
#6209=VERTEX_POINT ( 'NONE', #13994 ) ;
#6223=CARTESIAN_POINT ( 'NONE',  ( -35.00000000000000000, 17.00000000000000000, 39.00000000000003553 ) ) ;
#6240=EDGE_CURVE ( 'NONE', #15452, #17708, #21350, .T. ) ;
#6253=CARTESIAN_POINT ( 'NONE',  ( 35.00000000000000000, 10.00000000000000000, -40.99999999999997868 ) ) ;
#6254=ORIENTED_EDGE ( 'NONE', *, *, #8021, .F. ) ;
#6264=ORIENTED_EDGE ( 'NONE', *, *, #21917, .T. ) ;
#6266=EDGE_CURVE ( 'NONE', #9062, #16838, #14181, .T. ) ;
#6267=ORIENTED_EDGE ( 'NONE', *, *, #12925, .T. ) ;
#6293=EDGE_LOOP ( 'NONE', ( #10660, #3420 ) ) ;
#6298=DIRECTION ( 'NONE',  ( -1.067522139062650671E-15, 0.000000000000000000, -1.000000000000000000 ) ) ;
#6360=VERTEX_POINT ( 'NONE', #11493 ) ;
#6381=ORIENTED_EDGE ( 'NONE', *, *, #15884, .F. ) ;
#6432=VECTOR ( 'NONE', #6881, 1000.000000000000000 ) ;
#6485=ORIENTED_EDGE ( 'NONE', *, *, #15815, .T. ) ;
#6494=CARTESIAN_POINT ( 'NONE',  ( 28.52469787935785561, 7.000000000000000000, 4.095854054471903538 ) ) ;
#6498=DIRECTION ( 'NONE',  ( 0.000000000000000000, -1.000000000000000000, 0.000000000000000000 ) ) ;
#6503=ORIENTED_EDGE ( 'NONE', *, *, #20630, .T. ) ;
#6509=CIRCLE ( 'NONE', #4687, 2.500000000000002220 ) ;
#6512=CARTESIAN_POINT ( 'NONE',  ( 47.83731665821556334, 10.00000000000000000, -38.93845529828706020 ) ) ;
#6514=DIRECTION ( 'NONE',  ( 0.000000000000000000, 0.000000000000000000, -1.000000000000000000 ) ) ;
#6548=ORIENTED_EDGE ( 'NONE', *, *, #14606, .F. ) ;
#6549=ADVANCED_FACE ( 'NONE', ( #3079 ), #4582, .T. ) ;
#6573=VERTEX_POINT ( 'NONE', #16937 ) ;
#6576=DIRECTION ( 'NONE',  ( -0.000000000000000000, -1.000000000000000000, -0.000000000000000000 ) ) ;
#6592=ORIENTED_EDGE ( 'NONE', *, *, #6645, .F. ) ;
#6597=EDGE_CURVE ( 'NONE', #4837, #21104, #12122, .T. ) ;
#6599=ORIENTED_EDGE ( 'NONE', *, *, #8202, .T. ) ;
#6601=ORIENTED_EDGE ( 'NONE', *, *, #8021, .T. ) ;
#6608=AXIS2_PLACEMENT_3D ( 'NONE', #18848, #20121, #14510 ) ;
#6609=CARTESIAN_POINT ( 'NONE',  ( 35.00000000000000000, 10.00000000000000000, 41.00000000000002132 ) ) ;
#6611=CARTESIAN_POINT ( 'NONE',  ( 28.52469787935786982, 7.000000000000000000, -4.095854054471906203 ) ) ;
#6619=LINE ( 'NONE', #12332, #14910 ) ;
#6645=EDGE_CURVE ( 'NONE', #21941, #21842, #14040, .T. ) ;
#6653=ORIENTED_EDGE ( 'NONE', *, *, #19285, .F. ) ;
#6655=ORIENTED_EDGE ( 'NONE', *, *, #18444, .T. ) ;
#6662=LINE ( 'NONE', #9974, #13839 ) ;
#6690=ORIENTED_EDGE ( 'NONE', *, *, #20419, .T. ) ;
#6706=FACE_OUTER_BOUND ( 'NONE', #13210, .T. ) ;
#6711=ORIENTED_EDGE ( 'NONE', *, *, #12855, .F. ) ;
#6725=FACE_BOUND ( 'NONE', #8721, .T. ) ;
#6743=AXIS2_PLACEMENT_3D ( 'NONE', #1641, #10865, #12066 ) ;
#6751=CARTESIAN_POINT ( 'NONE',  ( 42.50000000000000000, 10.00000000000000000, 47.49999999999999289 ) ) ;
#6760=CARTESIAN_POINT ( 'NONE',  ( -36.06598984771573413, 10.00000000000000000, 48.42385786802029912 ) ) ;
#6777=DIRECTION ( 'NONE',  ( 0.000000000000000000, -1.000000000000000000, 0.000000000000000000 ) ) ;
#6796=FACE_OUTER_BOUND ( 'NONE', #8539, .T. ) ;
#6802=ORIENTED_EDGE ( 'NONE', *, *, #6240, .F. ) ;
#6805=ADVANCED_FACE ( 'NONE', ( #19799 ), #14725, .T. ) ;
#6816=AXIS2_PLACEMENT_3D ( 'NONE', #5436, #19196, #10463 ) ;
#6829=AXIS2_PLACEMENT_3D ( 'NONE', #15245, #4743, #11711 ) ;
#6836=ORIENTED_EDGE ( 'NONE', *, *, #97, .F. ) ;
#6845=FACE_OUTER_BOUND ( 'NONE', #7681, .T. ) ;
#6858=CARTESIAN_POINT ( 'NONE',  ( -35.00000000000000000, 13.99999999999999822, 15.00000000000002132 ) ) ;
#6864=CARTESIAN_POINT ( 'NONE',  ( 42.49999999999998579, 10.00000000000000000, -47.49999999999997868 ) ) ;
#6867=AXIS2_PLACEMENT_3D ( 'NONE', #13399, #22025, #22256 ) ;
#6869=CARTESIAN_POINT ( 'NONE',  ( -42.49999999999996447, 7.000000000000000000, -45.00000000000000711 ) ) ;
#6871=DIRECTION ( 'NONE',  ( 0.000000000000000000, -0.000000000000000000, -1.000000000000000000 ) ) ;
#6881=DIRECTION ( 'NONE',  ( 0.000000000000000000, -1.000000000000000000, 0.000000000000000000 ) ) ;
#6885=ORIENTED_EDGE ( 'NONE', *, *, #17210, .F. ) ;
#6888=CIRCLE ( 'NONE', #9447, 2.500000000000002220 ) ;
#6906=CARTESIAN_POINT ( 'NONE',  ( 41.39271818392635538, 10.00000000000000000, 5.943569790512533757 ) ) ;
#6923=CONICAL_SURFACE ( 'NONE', #19372, 39.00000000000001421, 0.7853981633974447263 ) ;
#6936=EDGE_CURVE ( 'NONE', #21565, #6573, #2833, .T. ) ;
#6974=ORIENTED_EDGE ( 'NONE', *, *, #12885, .F. ) ;
#6981=DIRECTION ( 'NONE',  ( 0.000000000000000000, -0.000000000000000000, -1.000000000000000000 ) ) ;
#6991=VERTEX_POINT ( 'NONE', #11865 ) ;
#6996=ORIENTED_EDGE ( 'NONE', *, *, #21917, .F. ) ;
#7003=CARTESIAN_POINT ( 'NONE',  ( 0.000000000000000000, 7.000000000000000000, 0.000000000000000000 ) ) ;
#7046=CYLINDRICAL_SURFACE ( 'NONE', #20278, 2.500000000000002220 ) ;
#7056=ADVANCED_FACE ( 'NONE', ( #21040 ), #21149, .F. ) ;
#7061=DIRECTION ( 'NONE',  ( 0.000000000000000000, 0.000000000000000000, -1.000000000000000000 ) ) ;
#7066=FACE_OUTER_BOUND ( 'NONE', #14925, .T. ) ;
#7085=PRODUCT_DEFINITION_SHAPE ( 'NONE', 'NONE',  #12887 ) ;
#7090=EDGE_CURVE ( 'NONE', #1691, #19883, #20599, .T. ) ;
#7104=CARTESIAN_POINT ( 'NONE',  ( 35.00000000000000000, -15.00000000000000000, 15.00000000000002132 ) ) ;
#7132=DIRECTION ( 'NONE',  ( 0.000000000000000000, -1.000000000000000000, 0.000000000000000000 ) ) ;
#7142=DIRECTION ( 'NONE',  ( 0.000000000000000000, -1.000000000000000000, 0.000000000000000000 ) ) ;
#7146=DIRECTION ( 'NONE',  ( -0.000000000000000000, -1.000000000000000000, -0.000000000000000000 ) ) ;
#7151=CIRCLE ( 'NONE', #3877, 17.00000000000000000 ) ;
#7156=EDGE_LOOP ( 'NONE', ( #1457, #12012 ) ) ;
#7158=VECTOR ( 'NONE', #12878, 1000.000000000000000 ) ;
#7167=AXIS2_PLACEMENT_3D ( 'NONE', #16932, #10045, #20494 ) ;
#7183=ADVANCED_FACE ( 'NONE', ( #16092 ), #7285, .F. ) ;
#7192=CARTESIAN_POINT ( 'NONE',  ( -35.00000000000000711, 0.000000000000000000, -38.99999999999997868 ) ) ;
#7195=FACE_BOUND ( 'NONE', #14076, .T. ) ;
#7197=ADVANCED_FACE ( 'NONE', ( #9567 ), #11049, .F. ) ;
#7203=ORIENTED_EDGE ( 'NONE', *, *, #16597, .T. ) ;
#7223=EDGE_CURVE ( 'NONE', #8088, #13043, #22084, .T. ) ;
#7248=ORIENTED_EDGE ( 'NONE', *, *, #13670, .T. ) ;
#7256=LINE ( 'NONE', #18012, #13820 ) ;
#7278=VECTOR ( 'NONE', #17303, 1000.000000000000000 ) ;
#7281=ORIENTED_EDGE ( 'NONE', *, *, #594, .T. ) ;
#7283=ORIENTED_EDGE ( 'NONE', *, *, #18365, .T. ) ;
#7285=PLANE ( 'NONE',  #16206 ) ;
#7288=DIRECTION ( 'NONE',  ( 0.000000000000000000, 0.000000000000000000, -1.000000000000000000 ) ) ;
#7301=EDGE_CURVE ( 'NONE', #6991, #968, #7802, .T. ) ;
#7314=CARTESIAN_POINT ( 'NONE',  ( -35.00000000000000000, 0.000000000000000000, 41.00000000000002132 ) ) ;
#7319=DIRECTION ( 'NONE',  ( 0.000000000000000000, 0.000000000000000000, -1.000000000000000000 ) ) ;
#7323=EDGE_CURVE ( 'NONE', #6360, #3151, #6003, .T. ) ;
#7332=EDGE_LOOP ( 'NONE', ( #9773, #8300, #5096, #18585 ) ) ;
#7334=DIRECTION ( 'NONE',  ( -0.000000000000000000, 1.000000000000000000, -0.000000000000000000 ) ) ;
#7339=EDGE_CURVE ( 'NONE', #13337, #21842, #16893, .T. ) ;
#7353=DIRECTION ( 'NONE',  ( 0.000000000000000000, -1.000000000000000000, 0.000000000000000000 ) ) ;
#7355=VERTEX_POINT ( 'NONE', #10115 ) ;
#7358=EDGE_CURVE ( 'NONE', #20463, #10413, #19172, .T. ) ;
#7361=ORIENTED_EDGE ( 'NONE', *, *, #13952, .T. ) ;
#7375=DIRECTION ( 'NONE',  ( 0.000000000000000000, 0.000000000000000000, -1.000000000000000000 ) ) ;
#7387=LINE ( 'NONE', #9214, #2367 ) ;
#7395=ORIENTED_EDGE ( 'NONE', *, *, #5963, .T. ) ;
#7421=DIRECTION ( 'NONE',  ( 1.000000000000000000, 0.000000000000000000, 0.000000000000000000 ) ) ;
#7422=CARTESIAN_POINT ( 'NONE',  ( -42.49999999999996447, 7.000000000000000000, -54.00000000000000711 ) ) ;
#7465=DIRECTION ( 'NONE',  ( 0.000000000000000000, 0.000000000000000000, -1.000000000000000000 ) ) ;
#7474=CARTESIAN_POINT ( 'NONE',  ( -35.00000000000000000, 22.00000000000000355, 2.365113165210053967E-14 ) ) ;
#7475=DIRECTION ( 'NONE',  ( -0.000000000000000000, -1.000000000000000000, -0.000000000000000000 ) ) ;
#7481=DIRECTION ( 'NONE',  ( -0.1421319796954317316, 0.000000000000000000, 0.9898477157360406897 ) ) ;
#7488=VERTEX_POINT ( 'NONE', #2734 ) ;
#7503=EDGE_LOOP ( 'NONE', ( #7203, #6885, #14103, #4294 ) ) ;
#7514=PLANE ( 'NONE',  #5602 ) ;
#7526=AXIS2_PLACEMENT_3D ( 'NONE', #19057, #14207, #10652 ) ;
#7532=AXIS2_PLACEMENT_3D ( 'NONE', #21987, #14962, #8004 ) ;
#7540=VECTOR ( 'NONE', #20912, 1000.000000000000000 ) ;
#7543=ORIENTED_EDGE ( 'NONE', *, *, #17616, .T. ) ;
#7544=DIRECTION ( 'NONE',  ( 0.000000000000000000, 0.000000000000000000, -1.000000000000000000 ) ) ;
#7581=VECTOR ( 'NONE', #5988, 1000.000000000000000 ) ;
#7597=PLANE ( 'NONE',  #10097 ) ;
#7611=FACE_OUTER_BOUND ( 'NONE', #3258, .T. ) ;
#7627=ORIENTED_EDGE ( 'NONE', *, *, #14322, .F. ) ;
#7630=CIRCLE ( 'NONE', #10162, 41.00000000000000000 ) ;
#7632=LINE ( 'NONE', #14938, #21446 ) ;
#7657=ORIENTED_EDGE ( 'NONE', *, *, #18367, .F. ) ;
#7678=ORIENTED_EDGE ( 'NONE', *, *, #5597, .F. ) ;
#7681=EDGE_LOOP ( 'NONE', ( #9596, #20791, #6503, #4051 ) ) ;
#7688=FACE_OUTER_BOUND ( 'NONE', #12227, .T. ) ;
#7699=ORIENTED_EDGE ( 'NONE', *, *, #7908, .F. ) ;
#7709=CARTESIAN_POINT ( 'NONE',  ( -42.49999999999996447, 10.00000000000000000, -47.50000000000000711 ) ) ;
#7726=VECTOR ( 'NONE', #138, 1000.000000000000000 ) ;
#7759=DIRECTION ( 'NONE',  ( 1.000000000000000000, 0.000000000000000000, -0.000000000000000000 ) ) ;
#7764=ORIENTED_EDGE ( 'NONE', *, *, #9254, .T. ) ;
#7777=EDGE_LOOP ( 'NONE', ( #13651, #6267, #20305, #12890 ) ) ;
#7787=LINE ( 'NONE', #4246, #4495 ) ;
#7798=DIRECTION ( 'NONE',  ( 0.000000000000000000, 0.000000000000000000, -1.000000000000000000 ) ) ;
#7802=CIRCLE ( 'NONE', #3072, 17.00000000000000000 ) ;
#7812=CARTESIAN_POINT ( 'NONE',  ( 35.00000000000000000, 10.00000000000000000, -40.99999999999997868 ) ) ;
#7834=LINE ( 'NONE', #8290, #21693 ) ;
#7839=EDGE_CURVE ( 'NONE', #12263, #3967, #17906, .T. ) ;
#7848=DIRECTION ( 'NONE',  ( -0.000000000000000000, 1.000000000000000000, -0.000000000000000000 ) ) ;
#7878=DIRECTION ( 'NONE',  ( 0.000000000000000000, 0.000000000000000000, 1.000000000000000000 ) ) ;
#7879=CYLINDRICAL_SURFACE ( 'NONE', #5088, 17.00000000000000000 ) ;
#7882=FACE_OUTER_BOUND ( 'NONE', #13438, .T. ) ;
#7895=CARTESIAN_POINT ( 'NONE',  ( 42.49999999999998579, 10.00000000000000000, -47.49999999999997868 ) ) ;
#7898=AXIS2_PLACEMENT_3D ( 'NONE', #20149, #11319, #14734 ) ;
#7908=EDGE_CURVE ( 'NONE', #8405, #8747, #9312, .T. ) ;
#7939=LINE ( 'NONE', #4280, #14594 ) ;
#7940=CARTESIAN_POINT ( 'NONE',  ( -35.00000000000000000, 22.00000000000000355, 17.00000000000002487 ) ) ;
#7954=LINE ( 'NONE', #4176, #3948 ) ;
#7969=CIRCLE ( 'NONE', #6867, 2.500000000000002220 ) ;
#8004=DIRECTION ( 'NONE',  ( 0.000000000000000000, 0.000000000000000000, -1.000000000000000000 ) ) ;
#8012=CARTESIAN_POINT ( 'NONE',  ( 35.00000000000000000, 25.00000000000000000, 2.365113165210053967E-14 ) ) ;
#8017=DIRECTION ( 'NONE',  ( 0.000000000000000000, 0.000000000000000000, -1.000000000000000000 ) ) ;
#8021=EDGE_CURVE ( 'NONE', #8747, #8574, #18246, .T. ) ;
#8025=DIRECTION ( 'NONE',  ( 0.000000000000000000, -1.000000000000000000, 0.000000000000000000 ) ) ;
#8058=CARTESIAN_POINT ( 'NONE',  ( 35.00000000000000000, 14.00000000000000000, -38.99999999999997868 ) ) ;
#8082=ORIENTED_EDGE ( 'NONE', *, *, #16095, .T. ) ;
#8088=VERTEX_POINT ( 'NONE', #12150 ) ;
#8102=ORIENTED_EDGE ( 'NONE', *, *, #12330, .F. ) ;
#8109=FACE_OUTER_BOUND ( 'NONE', #267, .T. ) ;
#8124=DIRECTION ( 'NONE',  ( 0.000000000000000000, -1.000000000000000000, 0.000000000000000000 ) ) ;
#8131=ORIENTED_EDGE ( 'NONE', *, *, #8513, .T. ) ;
#8138=ORIENTED_EDGE ( 'NONE', *, *, #11870, .T. ) ;
#8158=ORIENTED_EDGE ( 'NONE', *, *, #7323, .T. ) ;
#8160=CARTESIAN_POINT ( 'NONE',  ( -35.00000000000000000, 17.00000000000000000, -40.99999999999997868 ) ) ;
#8170=ORIENTED_EDGE ( 'NONE', *, *, #14597, .T. ) ;
#8171=CARTESIAN_POINT ( 'NONE',  ( -42.50000000000000000, 10.00000000000000000, 47.49999999999999289 ) ) ;
#8191=CARTESIAN_POINT ( 'NONE',  ( 42.50000000000000000, 7.000000000000000000, 47.49999999999999289 ) ) ;
#8202=EDGE_CURVE ( 'NONE', #13043, #8088, #19032, .T. ) ;
#8208=ORIENTED_EDGE ( 'NONE', *, *, #4776, .T. ) ;
#8256=VECTOR ( 'NONE', #15816, 1000.000000000000114 ) ;
#8280=ORIENTED_EDGE ( 'NONE', *, *, #19742, .F. ) ;
#8286=EDGE_LOOP ( 'NONE', ( #6013, #22051, #6057, #15770 ) ) ;
#8290=CARTESIAN_POINT ( 'NONE',  ( -35.00000000000000000, 17.00000000000000000, -40.99999999999997868 ) ) ;
#8300=ORIENTED_EDGE ( 'NONE', *, *, #12855, .T. ) ;
#8301=CARTESIAN_POINT ( 'NONE',  ( -42.49999999999996447, 10.00000000000000000, -47.50000000000000711 ) ) ;
#8309=LINE ( 'NONE', #14551, #13102 ) ;
#8335=AXIS2_PLACEMENT_3D ( 'NONE', #13874, #8616, #20892 ) ;
#8337=DIRECTION ( 'NONE',  ( 0.000000000000000000, 0.000000000000000000, -1.000000000000000000 ) ) ;
#8339=CIRCLE ( 'NONE', #19701, 6.499999999999999112 ) ;
#8357=CARTESIAN_POINT ( 'NONE',  ( 35.00000000000000000, 14.00000000000000000, -38.99999999999997868 ) ) ;
#8392=DIRECTION ( 'NONE',  ( -0.000000000000000000, 1.000000000000000000, -0.000000000000000000 ) ) ;
#8395=ORIENTED_EDGE ( 'NONE', *, *, #4776, .F. ) ;
#8405=VERTEX_POINT ( 'NONE', #693 ) ;
#8406=ORIENTED_EDGE ( 'NONE', *, *, #3162, .F. ) ;
#8420=AXIS2_PLACEMENT_3D ( 'NONE', #17261, #11062, #12778 ) ;
#8439=CARTESIAN_POINT ( 'NONE',  ( -41.39271818392636959, 7.000000000000000000, -5.943569790512535533 ) ) ;
#8459=VECTOR ( 'NONE', #5877, 1000.000000000000000 ) ;
#8473=( NAMED_UNIT ( * ) SI_UNIT ( $, .STERADIAN. ) SOLID_ANGLE_UNIT ( ) );
#8486=LINE ( 'NONE', #1844, #12128 ) ;
#8513=EDGE_CURVE ( 'NONE', #4381, #20633, #22229, .T. ) ;
#8537=FACE_OUTER_BOUND ( 'NONE', #17106, .T. ) ;
#8538=ORIENTED_EDGE ( 'NONE', *, *, #10471, .F. ) ;
#8539=EDGE_LOOP ( 'NONE', ( #6548, #3007, #17882, #15033 ) ) ;
#8574=VERTEX_POINT ( 'NONE', #12127 ) ;
#8577=DIRECTION ( 'NONE',  ( 0.000000000000000000, 0.000000000000000000, -1.000000000000000000 ) ) ;
#8582=EDGE_LOOP ( 'NONE', ( #1464, #12970, #11471, #972 ) ) ;
#8587=ORIENTED_EDGE ( 'NONE', *, *, #14762, .F. ) ;
#8602=CARTESIAN_POINT ( 'NONE',  ( 35.00000000000000000, 25.00000000000000000, -16.99999999999997868 ) ) ;
#8604=ORIENTED_EDGE ( 'NONE', *, *, #3134, .T. ) ;
#8609=DIRECTION ( 'NONE',  ( 0.000000000000000000, -1.000000000000000000, 0.000000000000000000 ) ) ;
#8616=DIRECTION ( 'NONE',  ( -0.000000000000000000, 1.000000000000000000, -0.000000000000000000 ) ) ;
#8619=CIRCLE ( 'NONE', #12626, 39.00000000000000000 ) ;
#8659=VERTEX_POINT ( 'NONE', #5581 ) ;
#8680=FACE_OUTER_BOUND ( 'NONE', #15303, .T. ) ;
#8685=ADVANCED_FACE ( 'NONE', ( #5368, #13937 ), #15671, .F. ) ;
#8694=DIRECTION ( 'NONE',  ( -0.000000000000000000, -1.000000000000000000, -0.000000000000000000 ) ) ;
#8701=VECTOR ( 'NONE', #14278, 1000.000000000000114 ) ;
#8720=FACE_OUTER_BOUND ( 'NONE', #7777, .T. ) ;
#8721=EDGE_LOOP ( 'NONE', ( #6080, #17614 ) ) ;
#8741=CARTESIAN_POINT ( 'NONE',  ( -28.52469787935786982, 7.000000000000000000, -4.095854054471906203 ) ) ;
#8745=EDGE_CURVE ( 'NONE', #8887, #21941, #14274, .T. ) ;
#8747=VERTEX_POINT ( 'NONE', #6253 ) ;
#8753=LINE ( 'NONE', #19181, #15065 ) ;
#8762=EDGE_LOOP ( 'NONE', ( #6974, #21872 ) ) ;
#8763=DIRECTION ( 'NONE',  ( 0.000000000000000000, -1.000000000000000000, 0.000000000000000000 ) ) ;
#8774=ADVANCED_FACE ( 'NONE', ( #20231, #3041 ), #4653, .F. ) ;
#8795=DIRECTION ( 'NONE',  ( 1.000000000000000000, 0.000000000000000000, 0.000000000000000000 ) ) ;
#8804=EDGE_CURVE ( 'NONE', #9999, #20208, #20885, .T. ) ;
#8824=VERTEX_POINT ( 'NONE', #10011 ) ;
#8844=CARTESIAN_POINT ( 'NONE',  ( 28.52469787935786982, 10.00000000000000000, -4.095854054471906203 ) ) ;
#8847=VERTEX_POINT ( 'NONE', #1432 ) ;
#8887=VERTEX_POINT ( 'NONE', #16415 ) ;
#8892=EDGE_CURVE ( 'NONE', #3556, #6991, #1986, .T. ) ;
#8919=LINE ( 'NONE', #1934, #3168 ) ;
#8931=AXIS2_PLACEMENT_3D ( 'NONE', #22123, #2651, #1038 ) ;
#8942=LINE ( 'NONE', #20884, #20687 ) ;
#8967=DIRECTION ( 'NONE',  ( 0.000000000000000000, 0.000000000000000000, -1.000000000000000000 ) ) ;
#8980=VECTOR ( 'NONE', #3554, 1000.000000000000114 ) ;
#9057=VECTOR ( 'NONE', #16923, 1000.000000000000000 ) ;
#9060=LINE ( 'NONE', #16036, #1579 ) ;
#9062=VERTEX_POINT ( 'NONE', #11255 ) ;
#9063=DIRECTION ( 'NONE',  ( 0.000000000000000000, -1.000000000000000000, 0.000000000000000000 ) ) ;
#9064=VECTOR ( 'NONE', #22424, 999.9999999999998863 ) ;
#9070=DIRECTION ( 'NONE',  ( 0.000000000000000000, -1.000000000000000000, 0.000000000000000000 ) ) ;
#9084=DIRECTION ( 'NONE',  ( 0.000000000000000000, 1.000000000000000000, 0.000000000000000000 ) ) ;
#9107=CARTESIAN_POINT ( 'NONE',  ( -42.50000000000000000, 7.000000000000000000, 49.99999999999999289 ) ) ;
#9157=DIRECTION ( 'NONE',  ( 0.000000000000000000, -0.000000000000000000, 1.000000000000000000 ) ) ;
#9180=CARTESIAN_POINT ( 'NONE',  ( -41.39271818392631985, 10.00000000000000000, 5.943569790512528428 ) ) ;
#9191=CARTESIAN_POINT ( 'NONE',  ( 48.93401015228426587, 10.00000000000000000, 46.57614213197968667 ) ) ;
#9196=PLANE ( 'NONE',  #22624 ) ;
#9204=VERTEX_POINT ( 'NONE', #17198 ) ;
#9214=CARTESIAN_POINT ( 'NONE',  ( 35.00000000000000000, 17.00000000000000000, 39.00000000000003553 ) ) ;
#9217=ORIENTED_EDGE ( 'NONE', *, *, #12124, .F. ) ;
#9221=CARTESIAN_POINT ( 'NONE',  ( -35.00000000000000000, -15.00000000000000000, 2.255140518769849223E-14 ) ) ;
#9224=ORIENTED_EDGE ( 'NONE', *, *, #7839, .T. ) ;
#9254=EDGE_CURVE ( 'NONE', #20081, #18060, #4843, .T. ) ;
#9267=AXIS2_PLACEMENT_3D ( 'NONE', #2271, #16240, #7544 ) ;
#9276=ORIENTED_EDGE ( 'NONE', *, *, #13419, .F. ) ;
#9312=LINE ( 'NONE', #255, #7726 ) ;
#9342=EDGE_LOOP ( 'NONE', ( #10544, #22673, #11027, #13725 ) ) ;
#9361=VECTOR ( 'NONE', #17434, 1000.000000000000114 ) ;
#9364=AXIS2_PLACEMENT_3D ( 'NONE', #2247, #865, #16336 ) ;
#9370=DIRECTION ( 'NONE',  ( 0.000000000000000000, 0.000000000000000000, -1.000000000000000000 ) ) ;
#9371=CARTESIAN_POINT ( 'NONE',  ( -42.49999999999996447, 10.00000000000000000, -47.50000000000000711 ) ) ;
#9378=LINE ( 'NONE', #3694, #12269 ) ;
#9384=EDGE_CURVE ( 'NONE', #6209, #3991, #19835, .T. ) ;
#9390=EDGE_LOOP ( 'NONE', ( #15698, #21146 ) ) ;
#9429=CARTESIAN_POINT ( 'NONE',  ( 35.00000000000000000, 17.00000000000000000, 41.00000000000002132 ) ) ;
#9442=ORIENTED_EDGE ( 'NONE', *, *, #7223, .T. ) ;
#9446=ORIENTED_EDGE ( 'NONE', *, *, #4273, .F. ) ;
#9447=AXIS2_PLACEMENT_3D ( 'NONE', #6751, #10393, #10174 ) ;
#9448=VECTOR ( 'NONE', #9063, 1000.000000000000000 ) ;
#9449=CARTESIAN_POINT ( 'NONE',  ( -42.50000000000000000, 10.00000000000000000, 47.49999999999999289 ) ) ;
#9457=VERTEX_POINT ( 'NONE', #1032 ) ;
#9460=AXIS2_PLACEMENT_3D ( 'NONE', #4869, #4650, #9681 ) ;
#9462=AXIS2_PLACEMENT_3D ( 'NONE', #22093, #16579, #11191 ) ;
#9472=CYLINDRICAL_SURFACE ( 'NONE', #18609, 2.500000000000002220 ) ;
#9491=DIRECTION ( 'NONE',  ( 1.000000000000000000, -0.000000000000000000, -0.000000000000000000 ) ) ;
#9557=CIRCLE ( 'NONE', #19796, 41.00000000000000000 ) ;
#9563=ORIENTED_EDGE ( 'NONE', *, *, #18444, .F. ) ;
#9567=FACE_OUTER_BOUND ( 'NONE', #3832, .T. ) ;
#9580=DIRECTION ( 'NONE',  ( 0.000000000000000000, -1.000000000000000000, 0.000000000000000000 ) ) ;
#9583=EDGE_CURVE ( 'NONE', #11088, #13179, #17851, .T. ) ;
#9588=EDGE_CURVE ( 'NONE', #21565, #8405, #5372, .T. ) ;
#9596=ORIENTED_EDGE ( 'NONE', *, *, #19541, .F. ) ;
#9609=VERTEX_POINT ( 'NONE', #10731 ) ;
#9628=AXIS2_PLACEMENT_3D ( 'NONE', #5749, #18114, #7465 ) ;
#9637=ORIENTED_EDGE ( 'NONE', *, *, #4711, .F. ) ;
#9656=ORIENTED_EDGE ( 'NONE', *, *, #3871, .F. ) ;
#9678=ADVANCED_FACE ( 'NONE', ( #18304 ), #18759, .F. ) ;
#9681=DIRECTION ( 'NONE',  ( 0.000000000000000000, 0.000000000000000000, 1.000000000000000000 ) ) ;
#9695=VERTEX_POINT ( 'NONE', #17030 ) ;
#9715=CIRCLE ( 'NONE', #4604, 41.00000000000000000 ) ;
#9730=ORIENTED_EDGE ( 'NONE', *, *, #10283, .F. ) ;
#9742=EDGE_LOOP ( 'NONE', ( #17344, #1430, #8082, #11158 ) ) ;
#9755=EDGE_CURVE ( 'NONE', #20463, #20208, #18997, .T. ) ;
#9773=ORIENTED_EDGE ( 'NONE', *, *, #2653, .T. ) ;
#9777=DIRECTION ( 'NONE',  ( 0.000000000000000000, 0.000000000000000000, -1.000000000000000000 ) ) ;
#9796=VERTEX_POINT ( 'NONE', #18653 ) ;
#9801=AXIS2_PLACEMENT_3D ( 'NONE', #7709, #21344, #5643 ) ;
#9814=AXIS2_PLACEMENT_3D ( 'NONE', #20285, #22004, #6298 ) ;
#9822=LINE ( 'NONE', #6494, #4453 ) ;
#9831=EDGE_CURVE ( 'NONE', #12985, #15787, #10149, .T. ) ;
#9843=CARTESIAN_POINT ( 'NONE',  ( -42.49999999999996447, 10.00000000000000000, -45.00000000000000711 ) ) ;
#9889=DIRECTION ( 'NONE',  ( 0.000000000000000000, 0.000000000000000000, -1.000000000000000000 ) ) ;
#9910=ORIENTED_EDGE ( 'NONE', *, *, #19541, .T. ) ;
#9922=ORIENTED_EDGE ( 'NONE', *, *, #12807, .T. ) ;
#9942=EDGE_CURVE ( 'NONE', #21624, #10917, #12655, .T. ) ;
#9958=CARTESIAN_POINT ( 'NONE',  ( 42.49999999999998579, 10.00000000000000000, -49.99999999999997868 ) ) ;
#9974=CARTESIAN_POINT ( 'NONE',  ( -35.00000000000000711, 14.00000000000000000, -38.99999999999997868 ) ) ;
#9999=VERTEX_POINT ( 'NONE', #17828 ) ;
#10011=CARTESIAN_POINT ( 'NONE',  ( 36.06598984771573413, 7.000000000000000000, 48.42385786802029912 ) ) ;
#10015=AXIS2_PLACEMENT_3D ( 'NONE', #18418, #2737, #6054 ) ;
#10036=DIRECTION ( 'NONE',  ( 0.000000000000000000, -1.000000000000000000, 0.000000000000000000 ) ) ;
#10045=DIRECTION ( 'NONE',  ( 0.000000000000000000, 1.000000000000000000, 0.000000000000000000 ) ) ;
#10050=CARTESIAN_POINT ( 'NONE',  ( 35.00000000000000000, 17.00000000000000000, 2.365113165210053967E-14 ) ) ;
#10056=DIRECTION ( 'NONE',  ( 0.000000000000000000, -1.000000000000000000, 0.000000000000000000 ) ) ;
#10074=VECTOR ( 'NONE', #1755, 1000.000000000000114 ) ;
#10084=FACE_BOUND ( 'NONE', #398, .T. ) ;
#10085=ORIENTED_EDGE ( 'NONE', *, *, #5776, .F. ) ;
#10092=CARTESIAN_POINT ( 'NONE',  ( 35.00000000000000000, -15.00000000000000000, -14.99999999999997691 ) ) ;
#10097=AXIS2_PLACEMENT_3D ( 'NONE', #8058, #948, #21586 ) ;
#10101=ADVANCED_FACE ( 'NONE', ( #4320 ), #9472, .F. ) ;
#10104=DIRECTION ( 'NONE',  ( 0.1421319796954317316, 0.000000000000000000, -0.9898477157360406897 ) ) ;
#10115=CARTESIAN_POINT ( 'NONE',  ( -35.00000000000000000, 0.000000000000000000, 39.00000000000002132 ) ) ;
#10143=DIRECTION ( 'NONE',  ( 0.1421319796954317316, 0.000000000000000000, -0.9898477157360405787 ) ) ;
#10149=LINE ( 'NONE', #1460, #2482 ) ;
#10162=AXIS2_PLACEMENT_3D ( 'NONE', #12429, #292, #7288 ) ;
#10166=AXIS2_PLACEMENT_3D ( 'NONE', #11824, #3130, #10104 ) ;
#10173=DIRECTION ( 'NONE',  ( 0.1421319796954322034, 0.000000000000000000, -0.9898477157360405787 ) ) ;
#10174=DIRECTION ( 'NONE',  ( 0.000000000000000000, 0.000000000000000000, -1.000000000000000000 ) ) ;
#10181=DIRECTION ( 'NONE',  ( 0.000000000000000000, 0.000000000000000000, -1.000000000000000000 ) ) ;
#10188=DIRECTION ( 'NONE',  ( -0.000000000000000000, 1.000000000000000000, -0.000000000000000000 ) ) ;
#10200=AXIS2_PLACEMENT_3D ( 'NONE', #16236, #2268, #428 ) ;
#10238=FACE_OUTER_BOUND ( 'NONE', #15263, .T. ) ;
#10248=DIRECTION ( 'NONE',  ( 0.000000000000000000, 0.000000000000000000, 1.000000000000000000 ) ) ;
#10283=EDGE_CURVE ( 'NONE', #10917, #9062, #11853, .T. ) ;
#10324=FACE_BOUND ( 'NONE', #8582, .T. ) ;
#10332=EDGE_CURVE ( 'NONE', #13358, #8824, #8309, .T. ) ;
#10338=DIRECTION ( 'NONE',  ( 0.000000000000000000, 0.000000000000000000, -1.000000000000000000 ) ) ;
#10346=CARTESIAN_POINT ( 'NONE',  ( -42.49999999999996447, 10.00000000000000000, -54.00000000000000711 ) ) ;
#10361=CARTESIAN_POINT ( 'NONE',  ( 28.52469787935786982, 10.00000000000000000, -4.095854054471906203 ) ) ;
#10365=DIRECTION ( 'NONE',  ( 0.000000000000000000, 1.000000000000000000, 0.000000000000000000 ) ) ;
#10393=DIRECTION ( 'NONE',  ( 0.000000000000000000, -1.000000000000000000, 0.000000000000000000 ) ) ;
#10396=DIRECTION ( 'NONE',  ( -0.000000000000000000, -1.000000000000000000, -0.000000000000000000 ) ) ;
#10413=VERTEX_POINT ( 'NONE', #2076 ) ;
#10463=DIRECTION ( 'NONE',  ( 0.000000000000000000, 0.000000000000000000, 1.000000000000000000 ) ) ;
#10470=DIRECTION ( 'NONE',  ( 0.000000000000000000, -1.000000000000000000, 0.000000000000000000 ) ) ;
#10471=EDGE_CURVE ( 'NONE', #8574, #9695, #3455, .T. ) ;
#10509=DIRECTION ( 'NONE',  ( 0.000000000000000000, 0.000000000000000000, -1.000000000000000000 ) ) ;
#10544=ORIENTED_EDGE ( 'NONE', *, *, #14754, .F. ) ;
#10570=CARTESIAN_POINT ( 'NONE',  ( 42.49999999999998579, 7.000000000000000000, -44.99999999999997868 ) ) ;
#10581=CARTESIAN_POINT ( 'NONE',  ( 35.00000000000000000, 14.00000000000000000, -38.99999999999997868 ) ) ;
#10593=CARTESIAN_POINT ( 'NONE',  ( 35.00000000000000000, 22.00000000000000355, 2.365113165210053967E-14 ) ) ;
#10606=FACE_BOUND ( 'NONE', #12229, .T. ) ;
#10611=DIRECTION ( 'NONE',  ( 0.000000000000000000, -1.000000000000000000, 0.000000000000000000 ) ) ;
#10617=MANIFOLD_SOLID_BREP ( 'Move Face1', #19217 ) ;
#10619=PLANE ( 'NONE',  #21796 ) ;
#10644=DIRECTION ( 'NONE',  ( -0.1421319796954322034, 0.000000000000000000, -0.9898477157360405787 ) ) ;
#10650=ORIENTED_EDGE ( 'NONE', *, *, #22489, .F. ) ;
#10652=DIRECTION ( 'NONE',  ( 0.000000000000000000, 0.000000000000000000, -1.000000000000000000 ) ) ;
#10660=ORIENTED_EDGE ( 'NONE', *, *, #2470, .T. ) ;
#10685=VECTOR ( 'NONE', #8694, 1000.000000000000000 ) ;
#10699=DIRECTION ( 'NONE',  ( -0.000000000000000000, -1.000000000000000000, -0.000000000000000000 ) ) ;
#10703=AXIS2_PLACEMENT_3D ( 'NONE', #19328, #22668, #13912 ) ;
#10711=DIRECTION ( 'NONE',  ( -0.000000000000000000, 1.000000000000000000, -0.000000000000000000 ) ) ;
#10712=ADVANCED_FACE ( 'NONE', ( #16016 ), #22132, .T. ) ;
#10719=EDGE_CURVE ( 'NONE', #20208, #9999, #13679, .T. ) ;
#10731=CARTESIAN_POINT ( 'NONE',  ( -35.00000000000000000, 22.00000000000000711, 15.00000000000002132 ) ) ;
#10754=FACE_OUTER_BOUND ( 'NONE', #4695, .T. ) ;
#10775=ORIENTED_EDGE ( 'NONE', *, *, #22554, .F. ) ;
#10776=CIRCLE ( 'NONE', #15495, 2.500000000000002220 ) ;
#10783=CARTESIAN_POINT ( 'NONE',  ( 35.00000000000000000, 15.00000000000000000, 2.365113165210053967E-14 ) ) ;
#10797=DIRECTION ( 'NONE',  ( 0.000000000000000000, 1.000000000000000000, 0.000000000000000000 ) ) ;
#10808=DIRECTION ( 'NONE',  ( 1.000000000000000000, 0.000000000000000000, 0.000000000000000000 ) ) ;
#10816=DIRECTION ( 'NONE',  ( -0.000000000000000000, 1.000000000000000000, -0.000000000000000000 ) ) ;
#10837=ORIENTED_EDGE ( 'NONE', *, *, #19112, .T. ) ;
#10865=DIRECTION ( 'NONE',  ( 0.000000000000000000, -1.000000000000000000, 0.000000000000000000 ) ) ;
#10867=AXIS2_PLACEMENT_3D ( 'NONE', #15234, #11592, #940 ) ;
#10894=LINE ( 'NONE', #19501, #9361 ) ;
#10898=VECTOR ( 'NONE', #1317, 1000.000000000000000 ) ;
#10917=VERTEX_POINT ( 'NONE', #4750 ) ;
#10935=PRODUCT_DEFINITION_FORMATION_WITH_SPECIFIED_SOURCE ( 'ANY', '', #17518, .NOT_KNOWN. ) ;
#10937=FACE_OUTER_BOUND ( 'NONE', #18926, .T. ) ;
#10947=VERTEX_POINT ( 'NONE', #17315 ) ;
#10969=CARTESIAN_POINT ( 'NONE',  ( -42.50000000000000000, 10.00000000000000000, 44.99999999999999289 ) ) ;
#10984=ORIENTED_EDGE ( 'NONE', *, *, #2899, .T. ) ;
#11007=ADVANCED_FACE ( 'NONE', ( #12717 ), #5406, .T. ) ;
#11013=DIRECTION ( 'NONE',  ( -0.000000000000000000, 1.000000000000000000, -0.000000000000000000 ) ) ;
#11024=EDGE_LOOP ( 'NONE', ( #2767, #20545, #16513, #20118 ) ) ;
#11027=ORIENTED_EDGE ( 'NONE', *, *, #5005, .T. ) ;
#11049=CYLINDRICAL_SURFACE ( 'NONE', #20250, 39.00000000000000000 ) ;
#11060=ADVANCED_FACE ( 'NONE', ( #7688 ), #21787, .F. ) ;
#11062=DIRECTION ( 'NONE',  ( 0.000000000000000000, 1.000000000000000000, 0.000000000000000000 ) ) ;
#11071=DIRECTION ( 'NONE',  ( -0.000000000000000000, -1.000000000000000000, -0.000000000000000000 ) ) ;
#11088=VERTEX_POINT ( 'NONE', #11579 ) ;
#11120=EDGE_LOOP ( 'NONE', ( #8280, #4359, #6183, #8131 ) ) ;
#11129=FACE_OUTER_BOUND ( 'NONE', #19542, .T. ) ;
#11145=CARTESIAN_POINT ( 'NONE',  ( 35.00000000000000000, 17.00000000000000000, 41.00000000000002132 ) ) ;
#11158=ORIENTED_EDGE ( 'NONE', *, *, #1810, .T. ) ;
#11162=DIRECTION ( 'NONE',  ( 0.000000000000000000, 0.000000000000000000, -1.000000000000000000 ) ) ;
#11167=CIRCLE ( 'NONE', #15539, 39.00000000000000000 ) ;
#11169=ORIENTED_EDGE ( 'NONE', *, *, #4547, .F. ) ;
#11185=ORIENTED_EDGE ( 'NONE', *, *, #8892, .F. ) ;
#11186=AXIS2_PLACEMENT_3D ( 'NONE', #20386, #16367, #6514 ) ;
#11191=DIRECTION ( 'NONE',  ( 0.000000000000000000, 0.000000000000000000, -1.000000000000000000 ) ) ;
#11209=ORIENTED_EDGE ( 'NONE', *, *, #14998, .F. ) ;
#11214=ORIENTED_EDGE ( 'NONE', *, *, #16902, .F. ) ;
#11255=CARTESIAN_POINT ( 'NONE',  ( -35.00000000000000000, 15.00000000000000000, 41.00000000000002132 ) ) ;
#11269=DIRECTION ( 'NONE',  ( 0.000000000000000000, -1.000000000000000000, 0.000000000000000000 ) ) ;
#11281=AXIS2_PLACEMENT_3D ( 'NONE', #3380, #15728, #10338 ) ;
#11293=DIRECTION ( 'NONE',  ( 0.000000000000000000, -1.000000000000000000, 0.000000000000000000 ) ) ;
#11297=VECTOR ( 'NONE', #11653, 999.9999999999998863 ) ;
#11317=DIRECTION ( 'NONE',  ( -0.000000000000000000, -1.000000000000000000, -0.000000000000000000 ) ) ;
#11319=DIRECTION ( 'NONE',  ( 0.000000000000000000, 0.7071067811865451302, 0.7071067811865500152 ) ) ;
#11388=ORIENTED_EDGE ( 'NONE', *, *, #4356, .T. ) ;
#11405=CARTESIAN_POINT ( 'NONE',  ( -35.00000000000000711, 14.00000000000000000, -38.99999999999997868 ) ) ;
#11410=LINE ( 'NONE', #14948, #6093 ) ;
#11425=CARTESIAN_POINT ( 'NONE',  ( -35.00000000000000000, 14.00000000000000000, 39.00000000000002132 ) ) ;
#11468=EDGE_CURVE ( 'NONE', #5292, #16920, #4180, .T. ) ;
#11471=ORIENTED_EDGE ( 'NONE', *, *, #2899, .F. ) ;
#11491=ORIENTED_EDGE ( 'NONE', *, *, #14660, .T. ) ;
#11493=CARTESIAN_POINT ( 'NONE',  ( -35.00000000000000000, 17.00000000000000000, -16.99999999999997868 ) ) ;
#11498=EDGE_LOOP ( 'NONE', ( #3052, #2815, #360, #21297 ) ) ;
#11502=FACE_OUTER_BOUND ( 'NONE', #13395, .T. ) ;
#11509=ORIENTED_EDGE ( 'NONE', *, *, #18187, .T. ) ;
#11510=ADVANCED_FACE ( 'NONE', ( #4116 ), #12908, .T. ) ;
#11515=ORIENTED_EDGE ( 'NONE', *, *, #5798, .F. ) ;
#11531=AXIS2_PLACEMENT_3D ( 'NONE', #9449, #11269, #4409 ) ;
#11568=ADVANCED_FACE ( 'NONE', ( #6706, #3625 ), #19201, .F. ) ;
#11569=LINE ( 'NONE', #18555, #1921 ) ;
#11579=CARTESIAN_POINT ( 'NONE',  ( -35.00000000000000000, 0.000000000000000000, 41.00000000000002132 ) ) ;
#11592=DIRECTION ( 'NONE',  ( 0.000000000000000000, -1.000000000000000000, 0.000000000000000000 ) ) ;
#11613=CARTESIAN_POINT ( 'NONE',  ( -28.52469787935782364, 10.00000000000000000, 4.095854054471899985 ) ) ;
#11620=ORIENTED_EDGE ( 'NONE', *, *, #10332, .F. ) ;
#11623=DIRECTION ( 'NONE',  ( 0.000000000000000000, 0.000000000000000000, -1.000000000000000000 ) ) ;
#11649=CARTESIAN_POINT ( 'NONE',  ( 42.49999999999998579, 10.00000000000000000, -44.99999999999997868 ) ) ;
#11653=DIRECTION ( 'NONE',  ( 0.1421319796954322034, 0.000000000000000000, 0.9898477157360405787 ) ) ;
#11658=AXIS2_PLACEMENT_3D ( 'NONE', #10593, #10365, #17249 ) ;
#11660=ORIENTED_EDGE ( 'NONE', *, *, #12555, .T. ) ;
#11667=DIRECTION ( 'NONE',  ( 0.000000000000000000, -1.000000000000000000, 0.000000000000000000 ) ) ;
#11693=CARTESIAN_POINT ( 'NONE',  ( 35.00000000000000000, 0.000000000000000000, -38.99999999999997868 ) ) ;
#11711=DIRECTION ( 'NONE',  ( 0.000000000000000000, 0.000000000000000000, 1.000000000000000000 ) ) ;
#11733=CARTESIAN_POINT ( 'NONE',  ( -35.00000000000000000, 17.00000000000000000, 2.365113165210053967E-14 ) ) ;
#11739=DIRECTION ( 'NONE',  ( -0.000000000000000000, -1.000000000000000000, -0.000000000000000000 ) ) ;
#11756=LINE ( 'NONE', #8439, #9064 ) ;
#11759=ORIENTED_EDGE ( 'NONE', *, *, #19972, .F. ) ;
#11760=CARTESIAN_POINT ( 'NONE',  ( -35.00000000000000000, 10.00000000000000000, 41.00000000000002132 ) ) ;
#11772=VERTEX_POINT ( 'NONE', #9107 ) ;
#11790=VECTOR ( 'NONE', #10173, 999.9999999999998863 ) ;
#11812=ORIENTED_EDGE ( 'NONE', *, *, #20217, .T. ) ;
#11813=CARTESIAN_POINT ( 'NONE',  ( 47.83731665821558465, 10.00000000000000000, 38.93845529828710283 ) ) ;
#11816=DIRECTION ( 'NONE',  ( -0.000000000000000000, 1.000000000000000000, -0.000000000000000000 ) ) ;
#11820=ORIENTED_EDGE ( 'NONE', *, *, #14998, .T. ) ;
#11824=CARTESIAN_POINT ( 'NONE',  ( -28.52469787935786982, 10.00000000000000000, -4.095854054471906203 ) ) ;
#11825=CARTESIAN_POINT ( 'NONE',  ( 35.00000000000000000, 7.000000000000000000, 2.365113165210053967E-14 ) ) ;
#11833=EDGE_LOOP ( 'NONE', ( #5993, #13240 ) ) ;
#11853=LINE ( 'NONE', #13665, #10898 ) ;
#11861=ORIENTED_EDGE ( 'NONE', *, *, #9583, .T. ) ;
#11862=( GEOMETRIC_REPRESENTATION_CONTEXT ( 3 ) GLOBAL_UNCERTAINTY_ASSIGNED_CONTEXT ( ( #16516 ) ) GLOBAL_UNIT_ASSIGNED_CONTEXT ( ( #20740, #1488, #8473 ) ) REPRESENTATION_CONTEXT ( 'NONE', 'WORKASPACE' ) );
#11865=CARTESIAN_POINT ( 'NONE',  ( 35.00000000000000000, 17.00000000000000000, 17.00000000000002487 ) ) ;
#11870=EDGE_CURVE ( 'NONE', #16838, #8887, #7834, .T. ) ;
#11877=ORIENTED_EDGE ( 'NONE', *, *, #10719, .T. ) ;
#11888=AXIS2_PLACEMENT_3D ( 'NONE', #13525, #20203, #18476 ) ;
#11890=ADVANCED_FACE ( 'NONE', ( #11502 ), #4638, .F. ) ;
#11904=CARTESIAN_POINT ( 'NONE',  ( -35.00000000000000000, 10.00000000000000000, 2.365113165210053967E-14 ) ) ;
#11918=SHAPE_DEFINITION_REPRESENTATION ( #7085, #15726 ) ;
#11934=ORIENTED_EDGE ( 'NONE', *, *, #19285, .T. ) ;
#11942=CIRCLE ( 'NONE', #19637, 2.500000000000002220 ) ;
#11967=CARTESIAN_POINT ( 'NONE',  ( -42.50000000000000000, 7.000000000000000000, 44.99999999999999289 ) ) ;
#12012=ORIENTED_EDGE ( 'NONE', *, *, #15136, .T. ) ;
#12016=AXIS2_PLACEMENT_3D ( 'NONE', #17485, #20937, #15411 ) ;
#12022=LINE ( 'NONE', #8357, #10685 ) ;
#12033=AXIS2_PLACEMENT_3D ( 'NONE', #13464, #6498, #22549 ) ;
#12058=LINE ( 'NONE', #4749, #17797 ) ;
#12064=CYLINDRICAL_SURFACE ( 'NONE', #7526, 39.00000000000000000 ) ;
#12066=DIRECTION ( 'NONE',  ( 0.000000000000000000, -0.000000000000000000, -1.000000000000000000 ) ) ;
#12084=CARTESIAN_POINT ( 'NONE',  ( -35.00000000000000000, 17.00000000000000000, 2.365113165210053967E-14 ) ) ;
#12093=CARTESIAN_POINT ( 'NONE',  ( -35.00000000000000000, 22.00000000000000711, 2.255140518769849223E-14 ) ) ;
#12097=EDGE_LOOP ( 'NONE', ( #17356, #13161, #5899, #20891 ) ) ;
#12105=ORIENTED_EDGE ( 'NONE', *, *, #15621, .T. ) ;
#12122=LINE ( 'NONE', #1821, #146 ) ;
#12124=EDGE_CURVE ( 'NONE', #4381, #13358, #21728, .T. ) ;
#12127=CARTESIAN_POINT ( 'NONE',  ( 35.00000000000000000, 6.999999999999999112, -40.99999999999997868 ) ) ;
#12128=VECTOR ( 'NONE', #13615, 1000.000000000000000 ) ;
#12150=CARTESIAN_POINT ( 'NONE',  ( -35.00000000000000000, 13.99999999999999822, -14.99999999999997691 ) ) ;
#12158=EDGE_CURVE ( 'NONE', #21624, #21565, #2314, .T. ) ;
#12173=ORIENTED_EDGE ( 'NONE', *, *, #13952, .F. ) ;
#12210=AXIS2_PLACEMENT_3D ( 'NONE', #4716, #4598, #20177 ) ;
#12214=EDGE_LOOP ( 'NONE', ( #19722, #11620, #628, #2320 ) ) ;
#12220=EDGE_CURVE ( 'NONE', #16743, #1869, #14004, .T. ) ;
#12227=EDGE_LOOP ( 'NONE', ( #16247, #18666, #18203, #20393 ) ) ;
#12229=EDGE_LOOP ( 'NONE', ( #12765, #18093 ) ) ;
#12240=LINE ( 'NONE', #19245, #8980 ) ;
#12263=VERTEX_POINT ( 'NONE', #12943 ) ;
#12269=VECTOR ( 'NONE', #10644, 999.9999999999998863 ) ;
#12270=CARTESIAN_POINT ( 'NONE',  ( -35.00000000000000000, 25.00000000000000000, 17.00000000000002487 ) ) ;
#12273=VERTEX_POINT ( 'NONE', #6088 ) ;
#12291=ORIENTED_EDGE ( 'NONE', *, *, #7090, .F. ) ;
#12304=AXIS2_PLACEMENT_3D ( 'NONE', #11904, #18909, #10181 ) ;
#12312=DIRECTION ( 'NONE',  ( 0.000000000000000000, 1.000000000000000000, 0.000000000000000000 ) ) ;
#12329=CIRCLE ( 'NONE', #12341, 15.00000000000000000 ) ;
#12330=EDGE_CURVE ( 'NONE', #15787, #9204, #816, .T. ) ;
#12332=CARTESIAN_POINT ( 'NONE',  ( 35.00000000000000000, 15.00000000000000000, -40.99999999999997868 ) ) ;
#12341=AXIS2_PLACEMENT_3D ( 'NONE', #17626, #1932, #15892 ) ;
#12348=FACE_OUTER_BOUND ( 'NONE', #11120, .T. ) ;
#12351=FACE_OUTER_BOUND ( 'NONE', #9742, .T. ) ;
#12353=EDGE_LOOP ( 'NONE', ( #20495, #14662, #11759, #13647 ) ) ;
#12405=CARTESIAN_POINT ( 'NONE',  ( -41.39271818392631985, 10.00000000000000000, 5.943569790512528428 ) ) ;
#12427=AXIS2_PLACEMENT_3D ( 'NONE', #3069, #20712, #8337 ) ;
#12429=CARTESIAN_POINT ( 'NONE',  ( 35.00000000000000000, 10.00000000000000000, 2.365113165210053967E-14 ) ) ;
#12431=ORIENTED_EDGE ( 'NONE', *, *, #12220, .T. ) ;
#12442=DIRECTION ( 'NONE',  ( 0.000000000000000000, -1.000000000000000000, 0.000000000000000000 ) ) ;
#12473=DIRECTION ( 'NONE',  ( -0.000000000000000000, 1.000000000000000000, -0.000000000000000000 ) ) ;
#12488=DIRECTION ( 'NONE',  ( 0.000000000000000000, 0.000000000000000000, -1.000000000000000000 ) ) ;
#12532=CARTESIAN_POINT ( 'NONE',  ( -35.00000000000000000, 14.00000000000000000, 2.365113165210053967E-14 ) ) ;
#12547=FACE_OUTER_BOUND ( 'NONE', #6293, .T. ) ;
#12555=EDGE_CURVE ( 'NONE', #16284, #5849, #3797, .T. ) ;
#12578=AXIS2_PLACEMENT_3D ( 'NONE', #17867, #21305, #9157 ) ;
#12585=ORIENTED_EDGE ( 'NONE', *, *, #16592, .F. ) ;
#12595=AXIS2_PLACEMENT_3D ( 'NONE', #20383, #11667, #4906 ) ;
#12609=ORIENTED_EDGE ( 'NONE', *, *, #11870, .F. ) ;
#12626=AXIS2_PLACEMENT_3D ( 'NONE', #16051, #14320, #12488 ) ;
#12651=FACE_OUTER_BOUND ( 'NONE', #22252, .T. ) ;
#12654=CARTESIAN_POINT ( 'NONE',  ( 47.83731665821558465, 10.00000000000000000, 38.93845529828710994 ) ) ;
#12655=LINE ( 'NONE', #21159, #20801 ) ;
#12684=PLANE ( 'NONE',  #169 ) ;
#12693=CIRCLE ( 'NONE', #20763, 2.500000000000002220 ) ;
#12717=FACE_OUTER_BOUND ( 'NONE', #9342, .T. ) ;
#12722=CARTESIAN_POINT ( 'NONE',  ( 35.00000000000000000, 17.00000000000000000, 2.365113165210053967E-14 ) ) ;
#12752=DIRECTION ( 'NONE',  ( 0.000000000000000000, 0.000000000000000000, 1.000000000000000000 ) ) ;
#12765=ORIENTED_EDGE ( 'NONE', *, *, #20358, .F. ) ;
#12778=DIRECTION ( 'NONE',  ( 0.000000000000000000, -0.000000000000000000, 1.000000000000000000 ) ) ;
#12782=DIRECTION ( 'NONE',  ( 0.000000000000000000, -1.000000000000000000, 0.000000000000000000 ) ) ;
#12807=EDGE_CURVE ( 'NONE', #9457, #21700, #2520, .T. ) ;
#12828=DIRECTION ( 'NONE',  ( -0.9898477157360405787, 0.000000000000000000, 0.1421319796954322312 ) ) ;
#12855=EDGE_CURVE ( 'NONE', #22631, #5849, #4355, .T. ) ;
#12878=DIRECTION ( 'NONE',  ( 0.000000000000000000, -1.000000000000000000, 0.000000000000000000 ) ) ;
#12885=EDGE_CURVE ( 'NONE', #15727, #16891, #963, .T. ) ;
#12887=PRODUCT_DEFINITION ( 'UNKNOWN', '', #10935, #2800 ) ;
#12890=ORIENTED_EDGE ( 'NONE', *, *, #6207, .F. ) ;
#12895=DIRECTION ( 'NONE',  ( 0.000000000000000000, 0.000000000000000000, -1.000000000000000000 ) ) ;
#12907=EDGE_CURVE ( 'NONE', #7488, #13097, #15575, .T. ) ;
#12908=CYLINDRICAL_SURFACE ( 'NONE', #16960, 17.00000000000000000 ) ;
#12925=EDGE_CURVE ( 'NONE', #9204, #3967, #13004, .T. ) ;
#12926=ORIENTED_EDGE ( 'NONE', *, *, #4433, .T. ) ;
#12943=CARTESIAN_POINT ( 'NONE',  ( -48.93401015228426587, 10.00000000000000000, 46.57614213197968667 ) ) ;
#12957=EDGE_CURVE ( 'NONE', #15034, #18483, #14487, .T. ) ;
#12970=ORIENTED_EDGE ( 'NONE', *, *, #19112, .F. ) ;
#12985=VERTEX_POINT ( 'NONE', #15423 ) ;
#12990=DIRECTION ( 'NONE',  ( 0.1421319796954322312, 0.000000000000000000, -0.9898477157360405787 ) ) ;
#13004=CIRCLE ( 'NONE', #11186, 6.499999999999999112 ) ;
#13006=CARTESIAN_POINT ( 'NONE',  ( -36.06598984771569860, 7.000000000000000000, -48.42385786802031333 ) ) ;
#13017=EDGE_CURVE ( 'NONE', #13636, #12273, #1470, .T. ) ;
#13020=DIRECTION ( 'NONE',  ( 0.000000000000000000, 1.000000000000000000, 0.000000000000000000 ) ) ;
#13033=EDGE_LOOP ( 'NONE', ( #9637, #6254, #21575, #5166 ) ) ;
#13035=VECTOR ( 'NONE', #8392, 1000.000000000000000 ) ;
#13043=VERTEX_POINT ( 'NONE', #6858 ) ;
#13059=ADVANCED_FACE ( 'NONE', ( #8680 ), #184, .T. ) ;
#13097=VERTEX_POINT ( 'NONE', #78 ) ;
#13100=DIRECTION ( 'NONE',  ( 0.000000000000000000, 0.000000000000000000, 1.000000000000000000 ) ) ;
#13102=VECTOR ( 'NONE', #9070, 1000.000000000000000 ) ;
#13105=DIRECTION ( 'NONE',  ( 0.000000000000000000, -1.000000000000000000, 0.000000000000000000 ) ) ;
#13108=ADVANCED_FACE ( 'NONE', ( #7066 ), #416, .F. ) ;
#13131=PLANE ( 'NONE',  #2431 ) ;
#13134=PLANE ( 'NONE',  #7898 ) ;
#13161=ORIENTED_EDGE ( 'NONE', *, *, #6936, .T. ) ;
#13179=VERTEX_POINT ( 'NONE', #21055 ) ;
#13210=EDGE_LOOP ( 'NONE', ( #20068, #21936, #4438, #16299, #14438 ) ) ;
#13233=CARTESIAN_POINT ( 'NONE',  ( -47.83731665821558465, 7.000000000000000000, 38.93845529828710283 ) ) ;
#13234=CARTESIAN_POINT ( 'NONE',  ( -35.00000000000000000, 25.00000000000000000, -16.99999999999997868 ) ) ;
#13237=DIRECTION ( 'NONE',  ( 0.000000000000000000, 0.7071067811865500152, 0.7071067811865451302 ) ) ;
#13240=ORIENTED_EDGE ( 'NONE', *, *, #359, .F. ) ;
#13243=DIRECTION ( 'NONE',  ( 0.000000000000000000, -1.000000000000000000, 0.000000000000000000 ) ) ;
#13247=EDGE_CURVE ( 'NONE', #57, #5656, #11410, .T. ) ;
#13248=AXIS2_PLACEMENT_3D ( 'NONE', #13671, #20686, #4995 ) ;
#13322=AXIS2_PLACEMENT_3D ( 'NONE', #9180, #12828, #19740 ) ;
#13331=AXIS2_PLACEMENT_3D ( 'NONE', #1575, #17498, #1814 ) ;
#13337=VERTEX_POINT ( 'NONE', #19898 ) ;
#13339=CARTESIAN_POINT ( 'NONE',  ( -35.00000000000000000, 17.00000000000000000, -38.99999999999999289 ) ) ;
#13347=LINE ( 'NONE', #1221, #11297 ) ;
#13350=CARTESIAN_POINT ( 'NONE',  ( 42.50000000000000000, 10.00000000000000000, 49.99999999999999289 ) ) ;
#13357=AXIS2_PLACEMENT_3D ( 'NONE', #3833, #10797, #17919 ) ;
#13358=VERTEX_POINT ( 'NONE', #19521 ) ;
#13370=DIRECTION ( 'NONE',  ( -0.000000000000000000, -1.000000000000000000, -0.000000000000000000 ) ) ;
#13389=APPLICATION_CONTEXT ( 'automotive_design' ) ;
#13395=EDGE_LOOP ( 'NONE', ( #18820, #6592, #3382, #20452 ) ) ;
#13399=CARTESIAN_POINT ( 'NONE',  ( -42.50000000000000000, 7.000000000000000000, 47.49999999999999289 ) ) ;
#13419=EDGE_CURVE ( 'NONE', #20633, #8824, #4293, .T. ) ;
#13433=AXIS2_PLACEMENT_3D ( 'NONE', #4961, #15138, #17209 ) ;
#13438=EDGE_LOOP ( 'NONE', ( #6802, #20190, #15718, #14963 ) ) ;
#13463=ORIENTED_EDGE ( 'NONE', *, *, #21253, .F. ) ;
#13464=CARTESIAN_POINT ( 'NONE',  ( 0.000000000000000000, 7.000000000000000000, 0.000000000000000000 ) ) ;
#13495=ORIENTED_EDGE ( 'NONE', *, *, #15621, .F. ) ;
#13508=ORIENTED_EDGE ( 'NONE', *, *, #10471, .T. ) ;
#13525=CARTESIAN_POINT ( 'NONE',  ( -35.00000000000000000, 0.000000000000000000, 2.365113165210053967E-14 ) ) ;
#13554=ORIENTED_EDGE ( 'NONE', *, *, #22211, .T. ) ;
#13615=DIRECTION ( 'NONE',  ( -0.000000000000000000, 1.000000000000000000, -0.000000000000000000 ) ) ;
#13636=VERTEX_POINT ( 'NONE', #18598 ) ;
#13642=VECTOR ( 'NONE', #1191, 1000.000000000000114 ) ;
#13643=FACE_OUTER_BOUND ( 'NONE', #22604, .T. ) ;
#13647=ORIENTED_EDGE ( 'NONE', *, *, #16444, .F. ) ;
#13651=ORIENTED_EDGE ( 'NONE', *, *, #16529, .T. ) ;
#13665=CARTESIAN_POINT ( 'NONE',  ( -35.00000000000000000, 15.00000000000000000, 41.00000000000002132 ) ) ;
#13668=STYLED_ITEM('',(#22748),#10617);
#13670=EDGE_CURVE ( 'NONE', #7488, #18483, #18819, .T. ) ;
#13671=CARTESIAN_POINT ( 'NONE',  ( 0.000000000000000000, 10.00000000000000000, 0.000000000000000000 ) ) ;
#13679=CIRCLE ( 'NONE', #9267, 2.500000000000002220 ) ;
#13691=DIRECTION ( 'NONE',  ( 0.000000000000000000, 0.000000000000000000, -1.000000000000000000 ) ) ;
#13705=EDGE_CURVE ( 'NONE', #14227, #22687, #15587, .T. ) ;
#13709=DIRECTION ( 'NONE',  ( 0.000000000000000000, 0.000000000000000000, -1.000000000000000000 ) ) ;
#13714=CARTESIAN_POINT ( 'NONE',  ( -35.00000000000000000, 14.00000000000000000, 39.00000000000002132 ) ) ;
#13725=ORIENTED_EDGE ( 'NONE', *, *, #13017, .T. ) ;
#13760=FACE_OUTER_BOUND ( 'NONE', #15772, .T. ) ;
#13783=ORIENTED_EDGE ( 'NONE', *, *, #14606, .T. ) ;
#13816=AXIS2_PLACEMENT_3D ( 'NONE', #6085, #11013, #7798 ) ;
#13820=VECTOR ( 'NONE', #17909, 1000.000000000000000 ) ;
#13839=VECTOR ( 'NONE', #13860, 1000.000000000000000 ) ;
#13848=CARTESIAN_POINT ( 'NONE',  ( -42.49999999999996447, 7.000000000000000000, -47.50000000000000711 ) ) ;
#13857=DIRECTION ( 'NONE',  ( 0.000000000000000000, -1.000000000000000000, 0.000000000000000000 ) ) ;
#13860=DIRECTION ( 'NONE',  ( -0.000000000000000000, -1.000000000000000000, -0.000000000000000000 ) ) ;
#13867=DIRECTION ( 'NONE',  ( 0.1421319796954322034, 0.000000000000000000, -0.9898477157360405787 ) ) ;
#13874=CARTESIAN_POINT ( 'NONE',  ( 42.49999999999998579, 7.000000000000000000, -47.49999999999997868 ) ) ;
#13912=DIRECTION ( 'NONE',  ( 0.000000000000000000, 0.000000000000000000, -1.000000000000000000 ) ) ;
#13928=CARTESIAN_POINT ( 'NONE',  ( -48.93401015228422324, 10.00000000000000000, -46.57614213197970088 ) ) ;
#13933=DIRECTION ( 'NONE',  ( 0.000000000000000000, -1.000000000000000000, 0.000000000000000000 ) ) ;
#13937=FACE_BOUND ( 'NONE', #11833, .T. ) ;
#13939=FACE_OUTER_BOUND ( 'NONE', #15594, .T. ) ;
#13952=EDGE_CURVE ( 'NONE', #19883, #11772, #22589, .T. ) ;
#13959=DIRECTION ( 'NONE',  ( 0.000000000000000000, -0.000000000000000000, -1.000000000000000000 ) ) ;
#13994=CARTESIAN_POINT ( 'NONE',  ( -47.83731665821558465, 10.00000000000000000, 38.93845529828710283 ) ) ;
#13998=LINE ( 'NONE', #10581, #17172 ) ;
#14004=CIRCLE ( 'NONE', #5596, 39.00000000000000000 ) ;
#14006=ORIENTED_EDGE ( 'NONE', *, *, #19445, .T. ) ;
#14008=AXIS2_PLACEMENT_3D ( 'NONE', #5910, #13105, #21380 ) ;
#14025=DIRECTION ( 'NONE',  ( 0.000000000000000000, -1.000000000000000000, 0.000000000000000000 ) ) ;
#14036=ORIENTED_EDGE ( 'NONE', *, *, #21253, .T. ) ;
#14040=LINE ( 'NONE', #15773, #1989 ) ;
#14054=DIRECTION ( 'NONE',  ( 0.1421319796954322034, 0.000000000000000000, 0.9898477157360405787 ) ) ;
#14076=EDGE_LOOP ( 'NONE', ( #6836, #19270 ) ) ;
#14103=ORIENTED_EDGE ( 'NONE', *, *, #18365, .F. ) ;
#14116=ORIENTED_EDGE ( 'NONE', *, *, #4356, .F. ) ;
#14153=VECTOR ( 'NONE', #15125, 1000.000000000000000 ) ;
#14175=AXIS2_PLACEMENT_3D ( 'NONE', #17362, #64, #5129 ) ;
#14181=CIRCLE ( 'NONE', #22278, 41.00000000000000000 ) ;
#14207=DIRECTION ( 'NONE',  ( -0.000000000000000000, -1.000000000000000000, -0.000000000000000000 ) ) ;
#14227=VERTEX_POINT ( 'NONE', #6512 ) ;
#14251=AXIS2_PLACEMENT_3D ( 'NONE', #3754, #10711, #17716 ) ;
#14263=AXIS2_PLACEMENT_3D ( 'NONE', #8191, #22177, #1096 ) ;
#14274=LINE ( 'NONE', #14937, #5153 ) ;
#14278=DIRECTION ( 'NONE',  ( 0.000000000000000000, -0.7071067811865500152, -0.7071067811865451302 ) ) ;
#14279=CARTESIAN_POINT ( 'NONE',  ( 0.000000000000000000, 7.000000000000000000, 0.000000000000000000 ) ) ;
#14317=ORIENTED_EDGE ( 'NONE', *, *, #20358, .T. ) ;
#14320=DIRECTION ( 'NONE',  ( 0.000000000000000000, -1.000000000000000000, 0.000000000000000000 ) ) ;
#14321=DIRECTION ( 'NONE',  ( 0.000000000000000000, 0.000000000000000000, -1.000000000000000000 ) ) ;
#14322=EDGE_CURVE ( 'NONE', #17708, #12273, #22514, .T. ) ;
#14369=ADVANCED_FACE ( 'NONE', ( #10606, #22564, #15767 ), #15658, .T. ) ;
#14392=CARTESIAN_POINT ( 'NONE',  ( 41.39271818392636959, 10.00000000000000000, -5.943569790512535533 ) ) ;
#14398=CARTESIAN_POINT ( 'NONE',  ( 42.49999999999998579, 10.00000000000000000, -47.49999999999997868 ) ) ;
#14416=VERTEX_POINT ( 'NONE', #3653 ) ;
#14438=ORIENTED_EDGE ( 'NONE', *, *, #13705, .T. ) ;
#14470=ADVANCED_FACE ( 'NONE', ( #10238 ), #20796, .T. ) ;
#14471=CIRCLE ( 'NONE', #17403, 2.500000000000002220 ) ;
#14487=CIRCLE ( 'NONE', #7167, 15.00000000000000000 ) ;
#14499=DIRECTION ( 'NONE',  ( 0.000000000000000000, 0.000000000000000000, -1.000000000000000000 ) ) ;
#14510=DIRECTION ( 'NONE',  ( 0.000000000000000000, -0.000000000000000000, -1.000000000000000000 ) ) ;
#14519=CARTESIAN_POINT ( 'NONE',  ( 35.00000000000000000, 14.00000000000000000, 2.365113165210053967E-14 ) ) ;
#14537=CIRCLE ( 'NONE', #9814, 6.499999999999999112 ) ;
#14551=CARTESIAN_POINT ( 'NONE',  ( 36.06598984771573413, 10.00000000000000000, 48.42385786802029912 ) ) ;
#14584=DIRECTION ( 'NONE',  ( 1.067522139062650671E-15, 0.000000000000000000, -1.000000000000000000 ) ) ;
#14594=VECTOR ( 'NONE', #20428, 999.9999999999998863 ) ;
#14597=EDGE_CURVE ( 'NONE', #8088, #19656, #16873, .T. ) ;
#14606=EDGE_CURVE ( 'NONE', #21700, #11088, #15543, .T. ) ;
#14607=ORIENTED_EDGE ( 'NONE', *, *, #19179, .F. ) ;
#14608=DIRECTION ( 'NONE',  ( 0.000000000000000000, -1.000000000000000000, 0.000000000000000000 ) ) ;
#14660=EDGE_CURVE ( 'NONE', #5292, #3151, #1744, .T. ) ;
#14662=ORIENTED_EDGE ( 'NONE', *, *, #13419, .T. ) ;
#14706=DIRECTION ( 'NONE',  ( 0.000000000000000000, 0.000000000000000000, -1.000000000000000000 ) ) ;
#14725=CYLINDRICAL_SURFACE ( 'NONE', #17717, 17.00000000000000000 ) ;
#14734=DIRECTION ( 'NONE',  ( -1.000000000000000000, 0.000000000000000000, 0.000000000000000000 ) ) ;
#14739=DIRECTION ( 'NONE',  ( 0.000000000000000000, -1.000000000000000000, 0.000000000000000000 ) ) ;
#14754=EDGE_CURVE ( 'NONE', #5656, #12273, #9378, .T. ) ;
#14762=EDGE_CURVE ( 'NONE', #10413, #9999, #8942, .T. ) ;
#14816=ADVANCED_FACE ( 'NONE', ( #20034 ), #13134, .T. ) ;
#14838=VECTOR ( 'NONE', #6180, 1000.000000000000000 ) ;
#14863=EDGE_CURVE ( 'NONE', #4837, #15126, #17766, .T. ) ;
#14886=ORIENTED_EDGE ( 'NONE', *, *, #5687, .F. ) ;
#14910=VECTOR ( 'NONE', #8795, 1000.000000000000000 ) ;
#14917=UNCERTAINTY_MEASURE_WITH_UNIT (LENGTH_MEASURE( 1.000000000000000082E-05 ), #4491, 'distance_accuracy_value', 'NONE');
#14925=EDGE_LOOP ( 'NONE', ( #4529, #10085, #3701, #18270 ) ) ;
#14935=ORIENTED_EDGE ( 'NONE', *, *, #21938, .T. ) ;
#14937=CARTESIAN_POINT ( 'NONE',  ( -28.52469787935782364, 10.00000000000000000, 4.095854054471899985 ) ) ;
#14938=CARTESIAN_POINT ( 'NONE',  ( 47.83731665821556334, 10.00000000000000000, -38.93845529828706020 ) ) ;
#14948=CARTESIAN_POINT ( 'NONE',  ( -47.83731665821552781, 10.00000000000000000, -38.93845529828706731 ) ) ;
#14962=DIRECTION ( 'NONE',  ( -0.000000000000000000, 1.000000000000000000, -0.000000000000000000 ) ) ;
#14963=ORIENTED_EDGE ( 'NONE', *, *, #20547, .T. ) ;
#14971=AXIS2_PLACEMENT_3D ( 'NONE', #2513, #13020, #2272 ) ;
#14998=EDGE_CURVE ( 'NONE', #3151, #6360, #7151, .T. ) ;
#15004=( NAMED_UNIT ( * ) SI_UNIT ( $, .STERADIAN. ) SOLID_ANGLE_UNIT ( ) );
#15025=FACE_OUTER_BOUND ( 'NONE', #21767, .T. ) ;
#15033=ORIENTED_EDGE ( 'NONE', *, *, #9583, .F. ) ;
#15034=VERTEX_POINT ( 'NONE', #18876 ) ;
#15065=VECTOR ( 'NONE', #5312, 1000.000000000000000 ) ;
#15081=DIRECTION ( 'NONE',  ( 0.000000000000000000, 0.000000000000000000, -1.000000000000000000 ) ) ;
#15096=AXIS2_PLACEMENT_3D ( 'NONE', #2237, #630, #11162 ) ;
#15125=DIRECTION ( 'NONE',  ( -0.000000000000000000, -1.000000000000000000, -0.000000000000000000 ) ) ;
#15126=VERTEX_POINT ( 'NONE', #21499 ) ;
#15136=EDGE_CURVE ( 'NONE', #19883, #1691, #14471, .T. ) ;
#15138=DIRECTION ( 'NONE',  ( 0.000000000000000000, -1.000000000000000000, 0.000000000000000000 ) ) ;
#15141=DIRECTION ( 'NONE',  ( 0.1421319796954317316, 0.000000000000000000, 0.9898477157360406897 ) ) ;
#15180=PLANE ( 'NONE',  #12033 ) ;
#15204=CARTESIAN_POINT ( 'NONE',  ( 35.00000000000000000, 17.00000000000000000, 39.00000000000003553 ) ) ;
#15210=CARTESIAN_POINT ( 'NONE',  ( 48.93401015228426587, 10.00000000000000000, 46.57614213197968667 ) ) ;
#15222=EDGE_CURVE ( 'NONE', #21941, #15452, #16306, .T. ) ;
#15234=CARTESIAN_POINT ( 'NONE',  ( 35.00000000000000000, 10.00000000000000000, 2.365113165210053967E-14 ) ) ;
#15245=CARTESIAN_POINT ( 'NONE',  ( -35.00000000000000000, 17.00000000000000000, 2.365113165210053967E-14 ) ) ;
#15256=CARTESIAN_POINT ( 'NONE',  ( -42.49999999999996447, 7.000000000000000000, -50.00000000000000711 ) ) ;
#15263=EDGE_LOOP ( 'NONE', ( #3938, #21688, #8208, #17954, #13783, #5536, #1013, #19118, #482, #18667, #16488, #8138 ) ) ;
#15271=CIRCLE ( 'NONE', #8335, 6.499999999999999112 ) ;
#15299=CARTESIAN_POINT ( 'NONE',  ( -36.06598984771569860, 10.00000000000000000, -48.42385786802031333 ) ) ;
#15301=DIRECTION ( 'NONE',  ( 1.000000000000000000, 0.000000000000000000, -0.000000000000000000 ) ) ;
#15303=EDGE_LOOP ( 'NONE', ( #9276, #16464, #18434, #5191 ) ) ;
#15378=VERTEX_POINT ( 'NONE', #11405 ) ;
#15411=DIRECTION ( 'NONE',  ( 0.000000000000000000, 0.000000000000000000, -1.000000000000000000 ) ) ;
#15423=CARTESIAN_POINT ( 'NONE',  ( -35.00000000000000000, 10.00000000000000000, 41.00000000000002132 ) ) ;
#15430=CYLINDRICAL_SURFACE ( 'NONE', #2485, 6.499999999999999112 ) ;
#15434=CARTESIAN_POINT ( 'NONE',  ( 41.39271818392635538, 7.000000000000000000, 5.943569790512533757 ) ) ;
#15452=VERTEX_POINT ( 'NONE', #10346 ) ;
#15476=CYLINDRICAL_SURFACE ( 'NONE', #608, 6.499999999999999112 ) ;
#15491=DIRECTION ( 'NONE',  ( 0.000000000000000000, 0.000000000000000000, 1.000000000000000000 ) ) ;
#15495=AXIS2_PLACEMENT_3D ( 'NONE', #19678, #5918, #14499 ) ;
#15534=ORIENTED_EDGE ( 'NONE', *, *, #16095, .F. ) ;
#15539=AXIS2_PLACEMENT_3D ( 'NONE', #14519, #5834, #4114 ) ;
#15543=CIRCLE ( 'NONE', #11888, 41.00000000000000000 ) ;
#15575=CIRCLE ( 'NONE', #18523, 15.00000000000000000 ) ;
#15579=PLANE ( 'NONE',  #2890 ) ;
#15582=CARTESIAN_POINT ( 'NONE',  ( 35.00000000000000000, 22.00000000000000355, -16.99999999999997868 ) ) ;
#15587=LINE ( 'NONE', #6906, #19662 ) ;
#15594=EDGE_LOOP ( 'NONE', ( #20296, #7678, #21453, #21609 ) ) ;
#15621=EDGE_CURVE ( 'NONE', #10947, #1869, #15838, .T. ) ;
#15632=VECTOR ( 'NONE', #7475, 1000.000000000000000 ) ;
#15649=DIRECTION ( 'NONE',  ( 0.000000000000000000, 0.000000000000000000, -1.000000000000000000 ) ) ;
#15652=ORIENTED_EDGE ( 'NONE', *, *, #5687, .T. ) ;
#15653=VECTOR ( 'NONE', #10470, 1000.000000000000000 ) ;
#15658=PLANE ( 'NONE',  #13331 ) ;
#15666=VECTOR ( 'NONE', #17142, 1000.000000000000114 ) ;
#15671=PLANE ( 'NONE',  #21618 ) ;
#15672=LINE ( 'NONE', #15434, #11790 ) ;
#15698=ORIENTED_EDGE ( 'NONE', *, *, #594, .F. ) ;
#15707=ADVANCED_FACE ( 'NONE', ( #4173 ), #21472, .F. ) ;
#15718=ORIENTED_EDGE ( 'NONE', *, *, #6645, .T. ) ;
#15726=SHAPE_REPRESENTATION ( 'REAR COVER', ( #18273 ), #22313 ) ;
#15727=VERTEX_POINT ( 'NONE', #9958 ) ;
#15728=DIRECTION ( 'NONE',  ( 0.000000000000000000, -1.000000000000000000, 0.000000000000000000 ) ) ;
#15735=DIRECTION ( 'NONE',  ( 0.000000000000000000, 0.000000000000000000, -1.000000000000000000 ) ) ;
#15767=FACE_OUTER_BOUND ( 'NONE', #12097, .T. ) ;
#15770=ORIENTED_EDGE ( 'NONE', *, *, #12330, .T. ) ;
#15772=EDGE_LOOP ( 'NONE', ( #12431, #13495, #15534, #18940 ) ) ;
#15773=CARTESIAN_POINT ( 'NONE',  ( -36.06598984771569860, 10.00000000000000000, -48.42385786802031333 ) ) ;
#15781=LINE ( 'NONE', #202, #17022 ) ;
#15787=VERTEX_POINT ( 'NONE', #6760 ) ;
#15815=EDGE_CURVE ( 'NONE', #57, #8887, #16685, .T. ) ;
#15816=DIRECTION ( 'NONE',  ( -0.1421319796954317316, 0.000000000000000000, 0.9898477157360405787 ) ) ;
#15825=DIRECTION ( 'NONE',  ( 0.000000000000000000, 0.000000000000000000, -1.000000000000000000 ) ) ;
#15838=LINE ( 'NONE', #19527, #2798 ) ;
#15878=ORIENTED_EDGE ( 'NONE', *, *, #22211, .F. ) ;
#15884=EDGE_CURVE ( 'NONE', #20081, #4381, #8919, .T. ) ;
#15890=FACE_OUTER_BOUND ( 'NONE', #3325, .T. ) ;
#15892=DIRECTION ( 'NONE',  ( 0.000000000000000000, 0.000000000000000000, 1.000000000000000000 ) ) ;
#15929=DIRECTION ( 'NONE',  ( -0.000000000000000000, -1.000000000000000000, -0.000000000000000000 ) ) ;
#16016=FACE_OUTER_BOUND ( 'NONE', #7503, .T. ) ;
#16036=CARTESIAN_POINT ( 'NONE',  ( -35.00000000000000000, 17.00000000000000000, 41.00000000000002132 ) ) ;
#16051=CARTESIAN_POINT ( 'NONE',  ( -35.00000000000000000, 14.00000000000000000, 2.365113165210053967E-14 ) ) ;
#16054=ADVANCED_FACE ( 'NONE', ( #552, #18077 ), #12684, .F. ) ;
#16071=CARTESIAN_POINT ( 'NONE',  ( 35.00000000000000000, 25.00000000000000000, 17.00000000000002487 ) ) ;
#16088=ORIENTED_EDGE ( 'NONE', *, *, #11468, .T. ) ;
#16090=ORIENTED_EDGE ( 'NONE', *, *, #9588, .F. ) ;
#16092=FACE_OUTER_BOUND ( 'NONE', #20714, .T. ) ;
#16095=EDGE_CURVE ( 'NONE', #8847, #10947, #11167, .T. ) ;
#16121=DIRECTION ( 'NONE',  ( 0.000000000000000000, -1.000000000000000000, 0.000000000000000000 ) ) ;
#16123=DIRECTION ( 'NONE',  ( 0.000000000000000000, -0.000000000000000000, -1.000000000000000000 ) ) ;
#16154=LINE ( 'NONE', #8741, #8256 ) ;
#16171=CARTESIAN_POINT ( 'NONE',  ( 28.52469787935785561, 10.00000000000000000, 4.095854054471903538 ) ) ;
#16189=ADVANCED_FACE ( 'NONE', ( #7611 ), #4295, .F. ) ;
#16197=EDGE_LOOP ( 'NONE', ( #4510, #7764, #18119, #13554, #6690, #20621, #13508, #20430, #21238, #7699, #11388, #16258 ) ) ;
#16206=AXIS2_PLACEMENT_3D ( 'NONE', #752, #14706, #17933 ) ;
#16231=DIRECTION ( 'NONE',  ( -0.1421319796954317316, 0.000000000000000000, -0.9898477157360405787 ) ) ;
#16236=CARTESIAN_POINT ( 'NONE',  ( -42.49999999999996447, 10.00000000000000000, -47.50000000000000711 ) ) ;
#16240=DIRECTION ( 'NONE',  ( 0.000000000000000000, -1.000000000000000000, 0.000000000000000000 ) ) ;
#16247=ORIENTED_EDGE ( 'NONE', *, *, #13670, .F. ) ;
#16258=ORIENTED_EDGE ( 'NONE', *, *, #4273, .T. ) ;
#16283=AXIS2_PLACEMENT_3D ( 'NONE', #14279, #19364, #6871 ) ;
#16284=VERTEX_POINT ( 'NONE', #15256 ) ;
#16299=ORIENTED_EDGE ( 'NONE', *, *, #4426, .T. ) ;
#16300=DIRECTION ( 'NONE',  ( 0.000000000000000000, -1.000000000000000000, 0.000000000000000000 ) ) ;
#16306=CIRCLE ( 'NONE', #9364, 6.499999999999999112 ) ;
#16336=DIRECTION ( 'NONE',  ( 1.067522139062650671E-15, 0.000000000000000000, -1.000000000000000000 ) ) ;
#16354=DIRECTION ( 'NONE',  ( 0.9898477157360405787, 0.000000000000000000, -0.1421319796954322312 ) ) ;
#16367=DIRECTION ( 'NONE',  ( 0.000000000000000000, -1.000000000000000000, 0.000000000000000000 ) ) ;
#16415=CARTESIAN_POINT ( 'NONE',  ( -35.00000000000000000, 10.00000000000000000, -40.99999999999997868 ) ) ;
#16416=FACE_OUTER_BOUND ( 'NONE', #11498, .T. ) ;
#16421=DIRECTION ( 'NONE',  ( 0.000000000000000000, -1.000000000000000000, 0.000000000000000000 ) ) ;
#16444=EDGE_CURVE ( 'NONE', #18060, #22660, #9715, .T. ) ;
#16454=ADVANCED_FACE ( 'NONE', ( #13760 ), #12064, .F. ) ;
#16464=ORIENTED_EDGE ( 'NONE', *, *, #8513, .F. ) ;
#16469=AXIS2_PLACEMENT_3D ( 'NONE', #16965, #13857, #5176 ) ;
#16473=ADVANCED_FACE ( 'NONE', ( #17895 ), #1861, .T. ) ;
#16488=ORIENTED_EDGE ( 'NONE', *, *, #6266, .T. ) ;
#16506=EDGE_CURVE ( 'NONE', #1054, #13358, #21220, .T. ) ;
#16513=ORIENTED_EDGE ( 'NONE', *, *, #7301, .T. ) ;
#16516=UNCERTAINTY_MEASURE_WITH_UNIT (LENGTH_MEASURE( 1.000000000000000082E-05 ), #20740, 'distance_accuracy_value', 'NONE');
#16526=ORIENTED_EDGE ( 'NONE', *, *, #20533, .T. ) ;
#16529=EDGE_CURVE ( 'NONE', #8659, #9204, #16154, .T. ) ;
#16579=DIRECTION ( 'NONE',  ( 0.000000000000000000, -1.000000000000000000, 0.000000000000000000 ) ) ;
#16592=EDGE_CURVE ( 'NONE', #5838, #15378, #8619, .T. ) ;
#16596=AXIS2_PLACEMENT_3D ( 'NONE', #13848, #10188, #1495 ) ;
#16597=EDGE_CURVE ( 'NONE', #9062, #17126, #10894, .T. ) ;
#16685=CIRCLE ( 'NONE', #12304, 41.00000000000000000 ) ;
#16739=CIRCLE ( 'NONE', #5410, 41.00000000000000000 ) ;
#16743=VERTEX_POINT ( 'NONE', #11693 ) ;
#16838=VERTEX_POINT ( 'NONE', #4675 ) ;
#16845=ADVANCED_FACE ( 'NONE', ( #8109 ), #2956, .F. ) ;
#16873=LINE ( 'NONE', #4846, #1283 ) ;
#16891=VERTEX_POINT ( 'NONE', #11649 ) ;
#16893=LINE ( 'NONE', #1091, #13642 ) ;
#16902=EDGE_CURVE ( 'NONE', #1054, #22660, #22325, .T. ) ;
#16918=AXIS2_PLACEMENT_3D ( 'NONE', #9221, #10816, #510 ) ;
#16920=VERTEX_POINT ( 'NONE', #21129 ) ;
#16923=DIRECTION ( 'NONE',  ( 0.000000000000000000, -1.000000000000000000, 0.000000000000000000 ) ) ;
#16932=CARTESIAN_POINT ( 'NONE',  ( 35.00000000000000000, 22.00000000000000711, 2.255140518769849223E-14 ) ) ;
#16937=CARTESIAN_POINT ( 'NONE',  ( -35.00000000000000000, 17.00000000000000000, -38.99999999999999289 ) ) ;
#16960=AXIS2_PLACEMENT_3D ( 'NONE', #8012, #4228, #18200 ) ;
#16965=CARTESIAN_POINT ( 'NONE',  ( -35.00000000000000000, 13.99999999999999822, 2.255140518769849223E-14 ) ) ;
#16993=DIRECTION ( 'NONE',  ( 1.000000000000000000, 0.000000000000000000, 0.000000000000000000 ) ) ;
#17022=VECTOR ( 'NONE', #10396, 1000.000000000000000 ) ;
#17026=DIRECTION ( 'NONE',  ( 0.000000000000000000, 0.000000000000000000, 1.000000000000000000 ) ) ;
#17030=CARTESIAN_POINT ( 'NONE',  ( 47.83731665821556334, 7.000000000000000000, -38.93845529828706020 ) ) ;
#17033=LINE ( 'NONE', #18659, #17935 ) ;
#17106=EDGE_LOOP ( 'NONE', ( #6711, #21268, #1265, #9563 ) ) ;
#17115=ADVANCED_FACE ( 'NONE', ( #16416 ), #7597, .F. ) ;
#17126=VERTEX_POINT ( 'NONE', #6223 ) ;
#17142=DIRECTION ( 'NONE',  ( 0.1421319796954317316, 0.000000000000000000, 0.9898477157360405787 ) ) ;
#17172=VECTOR ( 'NONE', #5329, 1000.000000000000000 ) ;
#17198=CARTESIAN_POINT ( 'NONE',  ( -36.06598984771573413, 7.000000000000000000, 48.42385786802029912 ) ) ;
#17209=DIRECTION ( 'NONE',  ( 0.000000000000000000, 0.000000000000000000, -1.000000000000000000 ) ) ;
#17210=EDGE_CURVE ( 'NONE', #6573, #17126, #21835, .T. ) ;
#17225=ORIENTED_EDGE ( 'NONE', *, *, #3623, .F. ) ;
#17249=DIRECTION ( 'NONE',  ( 0.000000000000000000, 0.000000000000000000, 1.000000000000000000 ) ) ;
#17261=CARTESIAN_POINT ( 'NONE',  ( 35.00000000000000000, 22.00000000000000355, 2.365113165210053967E-14 ) ) ;
#17303=DIRECTION ( 'NONE',  ( -0.000000000000000000, -1.000000000000000000, -0.000000000000000000 ) ) ;
#17315=CARTESIAN_POINT ( 'NONE',  ( 35.00000000000001421, 14.00000000000000000, 39.00000000000002132 ) ) ;
#17344=ORIENTED_EDGE ( 'NONE', *, *, #16592, .T. ) ;
#17356=ORIENTED_EDGE ( 'NONE', *, *, #12158, .T. ) ;
#17361=DIRECTION ( 'NONE',  ( -0.1421319796954317316, 0.000000000000000000, -0.9898477157360406897 ) ) ;
#17362=CARTESIAN_POINT ( 'NONE',  ( 35.00000000000000000, 22.00000000000000355, 2.365113165210053967E-14 ) ) ;
#17403=AXIS2_PLACEMENT_3D ( 'NONE', #3529, #14025, #7061 ) ;
#17434=DIRECTION ( 'NONE',  ( 0.000000000000000000, 0.7071067811865500152, -0.7071067811865451302 ) ) ;
#17485=CARTESIAN_POINT ( 'NONE',  ( 42.49999999999998579, 10.00000000000000000, -47.49999999999997868 ) ) ;
#17498=DIRECTION ( 'NONE',  ( 0.000000000000000000, 1.000000000000000000, 0.000000000000000000 ) ) ;
#17517=FACE_BOUND ( 'NONE', #2892, .T. ) ;
#17518=PRODUCT ( 'REAR COVER', 'REAR COVER', '', ( #1727 ) ) ;
#17553=DIRECTION ( 'NONE',  ( 0.000000000000000000, 0.000000000000000000, -1.000000000000000000 ) ) ;
#17556=ADVANCED_FACE ( 'NONE', ( #15890, #21070 ), #5160, .T. ) ;
#17614=ORIENTED_EDGE ( 'NONE', *, *, #10719, .F. ) ;
#17616=EDGE_CURVE ( 'NONE', #5838, #7355, #15781, .T. ) ;
#17626=CARTESIAN_POINT ( 'NONE',  ( 35.00000000000000000, 22.00000000000000711, 2.255140518769849223E-14 ) ) ;
#17655=EDGE_CURVE ( 'NONE', #8747, #15126, #12240, .T. ) ;
#17657=CARTESIAN_POINT ( 'NONE',  ( 35.00000000000000000, 25.00000000000000000, 2.365113165210053967E-14 ) ) ;
#17658=DIRECTION ( 'NONE',  ( 0.000000000000000000, 0.000000000000000000, 1.000000000000000000 ) ) ;
#17659=ADVANCED_FACE ( 'NONE', ( #7195, #17517, #12351 ), #10619, .T. ) ;
#17669=CARTESIAN_POINT ( 'NONE',  ( -48.93401015228426587, 10.00000000000000000, 46.57614213197968667 ) ) ;
#17693=ORIENTED_EDGE ( 'NONE', *, *, #9588, .T. ) ;
#17696=ORIENTED_EDGE ( 'NONE', *, *, #16506, .T. ) ;
#17698=CARTESIAN_POINT ( 'NONE',  ( -42.50000000000000000, 10.00000000000000000, 44.99999999999999289 ) ) ;
#17702=ADVANCED_FACE ( 'NONE', ( #7882 ), #19913, .T. ) ;
#17708=VERTEX_POINT ( 'NONE', #7422 ) ;
#17716=DIRECTION ( 'NONE',  ( 0.000000000000000000, 0.000000000000000000, -1.000000000000000000 ) ) ;
#17717=AXIS2_PLACEMENT_3D ( 'NONE', #4101, #11071, #9370 ) ;
#17723=ADVANCED_FACE ( 'NONE', ( #3305 ), #6923, .T. ) ;
#17735=DIRECTION ( 'NONE',  ( 0.000000000000000000, -1.000000000000000000, 0.000000000000000000 ) ) ;
#17746=CARTESIAN_POINT ( 'NONE',  ( -42.50000000000000000, 10.00000000000000000, 49.99999999999999289 ) ) ;
#17760=CARTESIAN_POINT ( 'NONE',  ( -35.00000000000000000, 17.00000000000000000, -38.99999999999999289 ) ) ;
#17766=CIRCLE ( 'NONE', #7532, 6.499999999999999112 ) ;
#17797=VECTOR ( 'NONE', #19053, 1000.000000000000000 ) ;
#17828=CARTESIAN_POINT ( 'NONE',  ( 42.50000000000000000, 7.000000000000000000, 44.99999999999999289 ) ) ;
#17851=LINE ( 'NONE', #7314, #3598 ) ;
#17860=CARTESIAN_POINT ( 'NONE',  ( 0.000000000000000000, 10.00000000000000000, 0.000000000000000000 ) ) ;
#17867=CARTESIAN_POINT ( 'NONE',  ( -35.00000000000000000, 0.000000000000000000, 2.365113165210053967E-14 ) ) ;
#17871=VECTOR ( 'NONE', #9491, 1000.000000000000000 ) ;
#17882=ORIENTED_EDGE ( 'NONE', *, *, #20419, .F. ) ;
#17895=FACE_OUTER_BOUND ( 'NONE', #11024, .T. ) ;
#17906=LINE ( 'NONE', #17669, #8459 ) ;
#17909=DIRECTION ( 'NONE',  ( -1.000000000000000000, -0.000000000000000000, -0.000000000000000000 ) ) ;
#17910=CARTESIAN_POINT ( 'NONE',  ( 36.06598984771572702, 10.00000000000000000, -48.42385786802028491 ) ) ;
#17919=DIRECTION ( 'NONE',  ( 0.000000000000000000, 0.000000000000000000, 1.000000000000000000 ) ) ;
#17933=DIRECTION ( 'NONE',  ( -1.000000000000000000, 0.000000000000000000, -0.000000000000000000 ) ) ;
#17935=VECTOR ( 'NONE', #13237, 1000.000000000000114 ) ;
#17954=ORIENTED_EDGE ( 'NONE', *, *, #5379, .T. ) ;
#17986=DIRECTION ( 'NONE',  ( 0.000000000000000000, 0.7071067811865451302, -0.7071067811865500152 ) ) ;
#18003=EDGE_CURVE ( 'NONE', #15378, #8847, #13998, .T. ) ;
#18012=CARTESIAN_POINT ( 'NONE',  ( -35.00000000000000000, 0.000000000000000000, 39.00000000000002132 ) ) ;
#18037=EDGE_LOOP ( 'NONE', ( #20022, #21974, #11877, #8587 ) ) ;
#18060=VERTEX_POINT ( 'NONE', #493 ) ;
#18077=FACE_OUTER_BOUND ( 'NONE', #4756, .T. ) ;
#18093=ORIENTED_EDGE ( 'NONE', *, *, #7301, .F. ) ;
#18114=DIRECTION ( 'NONE',  ( 0.000000000000000000, -1.000000000000000000, 0.000000000000000000 ) ) ;
#18119=ORIENTED_EDGE ( 'NONE', *, *, #16444, .T. ) ;
#18169=AXIS2_PLACEMENT_3D ( 'NONE', #7895, #1017, #8017 ) ;
#18187=EDGE_CURVE ( 'NONE', #19656, #9609, #716, .T. ) ;
#18189=LINE ( 'NONE', #13234, #2888 ) ;
#18192=CARTESIAN_POINT ( 'NONE',  ( 35.00000000000000000, 17.00000000000000000, 2.365113165210053967E-14 ) ) ;
#18195=DIRECTION ( 'NONE',  ( -0.000000000000000000, 1.000000000000000000, -0.000000000000000000 ) ) ;
#18200=DIRECTION ( 'NONE',  ( 0.000000000000000000, 0.000000000000000000, -1.000000000000000000 ) ) ;
#18203=ORIENTED_EDGE ( 'NONE', *, *, #22554, .T. ) ;
#18243=ORIENTED_EDGE ( 'NONE', *, *, #5233, .F. ) ;
#18246=LINE ( 'NONE', #7812, #4074 ) ;
#18270=ORIENTED_EDGE ( 'NONE', *, *, #8804, .T. ) ;
#18273=AXIS2_PLACEMENT_3D ( 'NONE', #1648, #15491, #16993 ) ;
#18296=VERTEX_POINT ( 'NONE', #1009 ) ;
#18304=FACE_OUTER_BOUND ( 'NONE', #809, .T. ) ;
#18351=LINE ( 'NONE', #1278, #336 ) ;
#18365=EDGE_CURVE ( 'NONE', #16838, #6573, #17033, .T. ) ;
#18367=EDGE_CURVE ( 'NONE', #15787, #12263, #21223, .T. ) ;
#18388=CARTESIAN_POINT ( 'NONE',  ( 42.50000000000000000, 10.00000000000000000, 47.49999999999999289 ) ) ;
#18418=CARTESIAN_POINT ( 'NONE',  ( -35.00000000000000000, 22.00000000000000355, 2.365113165210053967E-14 ) ) ;
#18434=ORIENTED_EDGE ( 'NONE', *, *, #12124, .T. ) ;
#18439=CARTESIAN_POINT ( 'NONE',  ( 42.49999999999998579, 7.000000000000000000, -47.49999999999997868 ) ) ;
#18444=EDGE_CURVE ( 'NONE', #5849, #16284, #21976, .T. ) ;
#18452=ADVANCED_FACE ( 'NONE', ( #21276, #12547 ), #3310, .T. ) ;
#18459=( NAMED_UNIT ( * ) PLANE_ANGLE_UNIT ( ) SI_UNIT ( $, .RADIAN. ) );
#18476=DIRECTION ( 'NONE',  ( 0.000000000000000000, 0.000000000000000000, 1.000000000000000000 ) ) ;
#18482=CARTESIAN_POINT ( 'NONE',  ( 42.49999999999998579, 7.000000000000000000, -47.49999999999997868 ) ) ;
#18483=VERTEX_POINT ( 'NONE', #19559 ) ;
#18494=ORIENTED_EDGE ( 'NONE', *, *, #4711, .T. ) ;
#18497=DIRECTION ( 'NONE',  ( 0.000000000000000000, 1.000000000000000000, 0.000000000000000000 ) ) ;
#18523=AXIS2_PLACEMENT_3D ( 'NONE', #18665, #8124, #15081 ) ;
#18555=CARTESIAN_POINT ( 'NONE',  ( 35.00000000000000000, 17.00000000000000000, -40.99999999999997868 ) ) ;
#18585=ORIENTED_EDGE ( 'NONE', *, *, #20237, .F. ) ;
#18594=ORIENTED_EDGE ( 'NONE', *, *, #5963, .F. ) ;
#18598=CARTESIAN_POINT ( 'NONE',  ( -48.93401015228422324, 10.00000000000000000, -46.57614213197970088 ) ) ;
#18609=AXIS2_PLACEMENT_3D ( 'NONE', #18388, #11293, #984 ) ;
#18653=CARTESIAN_POINT ( 'NONE',  ( 48.93401015228424455, 7.000000000000000000, -46.57614213197967956 ) ) ;
#18659=CARTESIAN_POINT ( 'NONE',  ( -35.00000000000000000, 15.00000000000000000, -40.99999999999997868 ) ) ;
#18665=CARTESIAN_POINT ( 'NONE',  ( 35.00000000000000000, 13.99999999999999822, 2.255140518769849223E-14 ) ) ;
#18666=ORIENTED_EDGE ( 'NONE', *, *, #12907, .T. ) ;
#18667=ORIENTED_EDGE ( 'NONE', *, *, #3134, .F. ) ;
#18676=CARTESIAN_POINT ( 'NONE',  ( -47.83731665821552781, 6.999999999999999112, -38.93845529828707441 ) ) ;
#18682=CARTESIAN_POINT ( 'NONE',  ( 42.49999999999998579, 7.000000000000000000, -53.99999999999997868 ) ) ;
#18759=CYLINDRICAL_SURFACE ( 'NONE', #21512, 2.500000000000002220 ) ;
#18782=CARTESIAN_POINT ( 'NONE',  ( -42.50000000000000000, 7.000000000000000000, 47.49999999999999289 ) ) ;
#18793=AXIS2_PLACEMENT_3D ( 'NONE', #12722, #468, #17658 ) ;
#18797=CIRCLE ( 'NONE', #14008, 41.00000000000000000 ) ;
#18816=DIRECTION ( 'NONE',  ( 0.000000000000000000, -1.000000000000000000, 0.000000000000000000 ) ) ;
#18819=LINE ( 'NONE', #10092, #13035 ) ;
#18820=ORIENTED_EDGE ( 'NONE', *, *, #7339, .T. ) ;
#18826=ORIENTED_EDGE ( 'NONE', *, *, #7908, .T. ) ;
#18837=ORIENTED_EDGE ( 'NONE', *, *, #20630, .F. ) ;
#18842=DIRECTION ( 'NONE',  ( 0.000000000000000000, 0.000000000000000000, 1.000000000000000000 ) ) ;
#18848=CARTESIAN_POINT ( 'NONE',  ( 0.000000000000000000, 10.00000000000000000, 0.000000000000000000 ) ) ;
#18876=CARTESIAN_POINT ( 'NONE',  ( 35.00000000000000000, 22.00000000000000711, 15.00000000000002132 ) ) ;
#18895=CIRCLE ( 'NONE', #4644, 6.499999999999999112 ) ;
#18901=CARTESIAN_POINT ( 'NONE',  ( 42.49999999999998579, 10.00000000000000000, -47.49999999999997868 ) ) ;
#18909=DIRECTION ( 'NONE',  ( 0.000000000000000000, -1.000000000000000000, 0.000000000000000000 ) ) ;
#18926=EDGE_LOOP ( 'NONE', ( #6599, #8170, #11509, #11169 ) ) ;
#18940=ORIENTED_EDGE ( 'NONE', *, *, #3808, .T. ) ;
#18943=CIRCLE ( 'NONE', #10867, 41.00000000000000000 ) ;
#18944=DIRECTION ( 'NONE',  ( 0.000000000000000000, 0.000000000000000000, -1.000000000000000000 ) ) ;
#18966=CYLINDRICAL_SURFACE ( 'NONE', #9462, 2.500000000000002220 ) ;
#18976=LINE ( 'NONE', #3507, #15653 ) ;
#18977=APPLICATION_CONTEXT ( 'automotive_design' ) ;
#18979=CIRCLE ( 'NONE', #13816, 2.500000000000002220 ) ;
#18981=CIRCLE ( 'NONE', #9460, 17.00000000000000000 ) ;
#18982=VECTOR ( 'NONE', #16300, 1000.000000000000000 ) ;
#18994=CARTESIAN_POINT ( 'NONE',  ( -42.50000000000000000, 10.00000000000000000, 49.99999999999999289 ) ) ;
#18997=LINE ( 'NONE', #13350, #9057 ) ;
#19032=CIRCLE ( 'NONE', #16469, 15.00000000000000000 ) ;
#19033=EDGE_CURVE ( 'NONE', #8887, #13337, #7954, .T. ) ;
#19053=DIRECTION ( 'NONE',  ( 0.000000000000000000, -1.000000000000000000, 0.000000000000000000 ) ) ;
#19057=CARTESIAN_POINT ( 'NONE',  ( 35.00000000000000000, 14.00000000000000000, 2.365113165210053967E-14 ) ) ;
#19072=CYLINDRICAL_SURFACE ( 'NONE', #11281, 2.500000000000002220 ) ;
#19112=EDGE_CURVE ( 'NONE', #7355, #3909, #1006, .T. ) ;
#19118=ORIENTED_EDGE ( 'NONE', *, *, #9384, .F. ) ;
#19120=AXIS2_PLACEMENT_3D ( 'NONE', #2351, #19437, #2124 ) ;
#19122=ORIENTED_EDGE ( 'NONE', *, *, #4999, .T. ) ;
#19172=CIRCLE ( 'NONE', #20612, 2.500000000000002220 ) ;
#19179=EDGE_CURVE ( 'NONE', #9796, #21104, #15271, .T. ) ;
#19181=CARTESIAN_POINT ( 'NONE',  ( -35.00000000000000000, 14.00000000000000000, 39.00000000000002132 ) ) ;
#19188=DIRECTION ( 'NONE',  ( 0.000000000000000000, -1.000000000000000000, 0.000000000000000000 ) ) ;
#19196=DIRECTION ( 'NONE',  ( 0.000000000000000000, 1.000000000000000000, 0.000000000000000000 ) ) ;
#19201=PLANE ( 'NONE',  #13248 ) ;
#19202=ADVANCED_FACE ( 'NONE', ( #1411 ), #4854, .T. ) ;
#19209=AXIS2_PLACEMENT_3D ( 'NONE', #328, #16121, #7319 ) ;
#19217=CLOSED_SHELL ( 'NONE', ( #22568, #1607, #10101, #2879, #21621, #6076, #5223, #16189, #16473, #6805, #6549, #14470, #7183, #16845, #14369, #855, #14816, #17723, #10712, #3482, #6107, #2070, #11510, #18452, #7197, #4010, #16454, #17115, #17659, #19202, #4841, #20611, #9678, #8774, #22414, #17702, #11007, #11890, #565, #8685, #807, #5820, #5245, #1632, #19876, #11568, #17556, #5924, #7056, #13108, #13059, #16054, #19819, #15707, #11060 ) ) ;
#19221=DIRECTION ( 'NONE',  ( 0.000000000000000000, 0.000000000000000000, 1.000000000000000000 ) ) ;
#19245=CARTESIAN_POINT ( 'NONE',  ( 28.52469787935785561, 10.00000000000000000, 4.095854054471903538 ) ) ;
#19264=VECTOR ( 'NONE', #20947, 1000.000000000000000 ) ;
#19270=ORIENTED_EDGE ( 'NONE', *, *, #12907, .F. ) ;
#19285=EDGE_CURVE ( 'NONE', #18296, #5024, #18979, .T. ) ;
#19294=ORIENTED_EDGE ( 'NONE', *, *, #12158, .F. ) ;
#19302=DIRECTION ( 'NONE',  ( -0.1421319796954322034, 0.000000000000000000, -0.9898477157360405787 ) ) ;
#19328=CARTESIAN_POINT ( 'NONE',  ( -42.50000000000000000, 10.00000000000000000, 47.49999999999999289 ) ) ;
#19347=CARTESIAN_POINT ( 'NONE',  ( 42.50000000000000000, 10.00000000000000000, 47.49999999999999289 ) ) ;
#19364=DIRECTION ( 'NONE',  ( 0.000000000000000000, -1.000000000000000000, 0.000000000000000000 ) ) ;
#19372=AXIS2_PLACEMENT_3D ( 'NONE', #18192, #5354, #13691 ) ;
#19437=DIRECTION ( 'NONE',  ( -0.9898477157360405787, 0.000000000000000000, -0.1421319796954322312 ) ) ;
#19445=EDGE_CURVE ( 'NONE', #16838, #8405, #6619, .T. ) ;
#19449=DIRECTION ( 'NONE',  ( 0.000000000000000000, -0.7071067811865500152, 0.7071067811865451302 ) ) ;
#19463=CARTESIAN_POINT ( 'NONE',  ( -48.93401015228426587, 7.000000000000000000, 46.57614213197968667 ) ) ;
#19501=CARTESIAN_POINT ( 'NONE',  ( -35.00000000000000000, 15.00000000000000000, 41.00000000000002132 ) ) ;
#19504=ORIENTED_EDGE ( 'NONE', *, *, #2637, .F. ) ;
#19521=CARTESIAN_POINT ( 'NONE',  ( 36.06598984771573413, 10.00000000000000000, 48.42385786802029912 ) ) ;
#19527=CARTESIAN_POINT ( 'NONE',  ( 35.00000000000001421, 14.00000000000000000, 39.00000000000002132 ) ) ;
#19531=AXIS2_PLACEMENT_3D ( 'NONE', #11733, #18497, #13100 ) ;
#19541=EDGE_CURVE ( 'NONE', #16891, #5024, #18976, .T. ) ;
#19542=EDGE_LOOP ( 'NONE', ( #3633, #16088 ) ) ;
#19559=CARTESIAN_POINT ( 'NONE',  ( 35.00000000000000000, 22.00000000000000711, -14.99999999999997691 ) ) ;
#19600=PLANE ( 'NONE',  #22445 ) ;
#19637=AXIS2_PLACEMENT_3D ( 'NONE', #18482, #2795, #9777 ) ;
#19646=CARTESIAN_POINT ( 'NONE',  ( 42.50000000000000000, 10.00000000000000000, 49.99999999999999289 ) ) ;
#19656=VERTEX_POINT ( 'NONE', #20746 ) ;
#19662=VECTOR ( 'NONE', #13867, 999.9999999999998863 ) ;
#19665=EDGE_LOOP ( 'NONE', ( #472, #6264, #3018, #6485, #22341 ) ) ;
#19678=CARTESIAN_POINT ( 'NONE',  ( -42.49999999999996447, 10.00000000000000000, -47.50000000000000711 ) ) ;
#19684=ORIENTED_EDGE ( 'NONE', *, *, #11468, .F. ) ;
#19701=AXIS2_PLACEMENT_3D ( 'NONE', #18439, #20608, #10509 ) ;
#19722=ORIENTED_EDGE ( 'NONE', *, *, #19972, .T. ) ;
#19736=ORIENTED_EDGE ( 'NONE', *, *, #19922, .T. ) ;
#19740=DIRECTION ( 'NONE',  ( 0.1421319796954322312, 0.000000000000000000, 0.9898477157360405787 ) ) ;
#19742=EDGE_CURVE ( 'NONE', #18060, #20633, #13347, .T. ) ;
#19749=DIRECTION ( 'NONE',  ( 0.000000000000000000, -0.000000000000000000, 1.000000000000000000 ) ) ;
#19796=AXIS2_PLACEMENT_3D ( 'NONE', #5318, #19188, #8967 ) ;
#19797=EDGE_LOOP ( 'NONE', ( #11185, #4526, #5666, #14317 ) ) ;
#19799=FACE_OUTER_BOUND ( 'NONE', #3196, .T. ) ;
#19819=ADVANCED_FACE ( 'NONE', ( #6725, #5132 ), #15180, .T. ) ;
#19835=LINE ( 'NONE', #2069, #9448 ) ;
#19847=ORIENTED_EDGE ( 'NONE', *, *, #9831, .F. ) ;
#19868=EDGE_LOOP ( 'NONE', ( #3632, #9730, #20041, #20160 ) ) ;
#19876=ADVANCED_FACE ( 'NONE', ( #6845 ), #4897, .F. ) ;
#19883=VERTEX_POINT ( 'NONE', #18994 ) ;
#19896=CIRCLE ( 'NONE', #5623, 15.00000000000000000 ) ;
#19898=CARTESIAN_POINT ( 'NONE',  ( -35.00000000000000000, 7.000000000000000000, -40.99999999999997868 ) ) ;
#19913=CYLINDRICAL_SURFACE ( 'NONE', #10200, 6.499999999999999112 ) ;
#19922=EDGE_CURVE ( 'NONE', #12985, #8659, #20587, .T. ) ;
#19972=EDGE_CURVE ( 'NONE', #22660, #8824, #22327, .T. ) ;
#20007=AXIS2_PLACEMENT_3D ( 'NONE', #19347, #12442, #3654 ) ;
#20022=ORIENTED_EDGE ( 'NONE', *, *, #7358, .F. ) ;
#20023=EDGE_LOOP ( 'NONE', ( #11660, #6655 ) ) ;
#20034=FACE_OUTER_BOUND ( 'NONE', #19868, .T. ) ;
#20041=ORIENTED_EDGE ( 'NONE', *, *, #9942, .F. ) ;
#20068=ORIENTED_EDGE ( 'NONE', *, *, #5597, .T. ) ;
#20081=VERTEX_POINT ( 'NONE', #12654 ) ;
#20118=ORIENTED_EDGE ( 'NONE', *, *, #3240, .F. ) ;
#20121=DIRECTION ( 'NONE',  ( 0.000000000000000000, -1.000000000000000000, 0.000000000000000000 ) ) ;
#20137=ORIENTED_EDGE ( 'NONE', *, *, #7839, .F. ) ;
#20141=DIRECTION ( 'NONE',  ( -0.000000000000000000, 1.000000000000000000, -0.000000000000000000 ) ) ;
#20149=CARTESIAN_POINT ( 'NONE',  ( -35.00000000000000000, 17.00000000000000000, 39.00000000000003553 ) ) ;
#20160=ORIENTED_EDGE ( 'NONE', *, *, #748, .F. ) ;
#20177=DIRECTION ( 'NONE',  ( 0.000000000000000000, 0.000000000000000000, 1.000000000000000000 ) ) ;
#20190=ORIENTED_EDGE ( 'NONE', *, *, #15222, .F. ) ;
#20203=DIRECTION ( 'NONE',  ( 0.000000000000000000, 1.000000000000000000, 0.000000000000000000 ) ) ;
#20208=VERTEX_POINT ( 'NONE', #639 ) ;
#20217=EDGE_CURVE ( 'NONE', #14227, #9695, #7632, .T. ) ;
#20225=DIRECTION ( 'NONE',  ( 0.000000000000000000, 1.000000000000000000, 0.000000000000000000 ) ) ;
#20231=FACE_OUTER_BOUND ( 'NONE', #3027, .T. ) ;
#20237=EDGE_CURVE ( 'NONE', #14416, #16284, #22067, .T. ) ;
#20250=AXIS2_PLACEMENT_3D ( 'NONE', #12532, #21263, #6016 ) ;
#20257=CARTESIAN_POINT ( 'NONE',  ( 35.00000000000000000, 0.000000000000000000, -38.99999999999997868 ) ) ;
#20278=AXIS2_PLACEMENT_3D ( 'NONE', #22534, #3626, #3509 ) ;
#20285=CARTESIAN_POINT ( 'NONE',  ( 42.49999999999998579, 10.00000000000000000, -47.49999999999997868 ) ) ;
#20296=ORIENTED_EDGE ( 'NONE', *, *, #6597, .F. ) ;
#20305=ORIENTED_EDGE ( 'NONE', *, *, #21938, .F. ) ;
#20358=EDGE_CURVE ( 'NONE', #968, #6991, #3535, .T. ) ;
#20383=CARTESIAN_POINT ( 'NONE',  ( 35.00000000000000000, 13.99999999999999822, 2.255140518769849223E-14 ) ) ;
#20386=CARTESIAN_POINT ( 'NONE',  ( -42.50000000000000000, 7.000000000000000000, 47.49999999999999289 ) ) ;
#20393=ORIENTED_EDGE ( 'NONE', *, *, #12957, .T. ) ;
#20419=EDGE_CURVE ( 'NONE', #13179, #9457, #1693, .T. ) ;
#20428=DIRECTION ( 'NONE',  ( -0.1421319796954322034, 0.000000000000000000, 0.9898477157360405787 ) ) ;
#20430=ORIENTED_EDGE ( 'NONE', *, *, #20217, .F. ) ;
#20452=ORIENTED_EDGE ( 'NONE', *, *, #19033, .T. ) ;
#20463=VERTEX_POINT ( 'NONE', #19646 ) ;
#20494=DIRECTION ( 'NONE',  ( 0.000000000000000000, 0.000000000000000000, 1.000000000000000000 ) ) ;
#20495=ORIENTED_EDGE ( 'NONE', *, *, #19742, .T. ) ;
#20533=EDGE_CURVE ( 'NONE', #5024, #18296, #11942, .T. ) ;
#20545=ORIENTED_EDGE ( 'NONE', *, *, #8892, .T. ) ;
#20547=EDGE_CURVE ( 'NONE', #21842, #17708, #18895, .T. ) ;
#20587=LINE ( 'NONE', #11760, #6181 ) ;
#20599=CIRCLE ( 'NONE', #10703, 2.500000000000002220 ) ;
#20608=DIRECTION ( 'NONE',  ( -0.000000000000000000, 1.000000000000000000, -0.000000000000000000 ) ) ;
#20611=ADVANCED_FACE ( 'NONE', ( #15025 ), #15476, .T. ) ;
#20612=AXIS2_PLACEMENT_3D ( 'NONE', #137, #7132, #15825 ) ;
#20621=ORIENTED_EDGE ( 'NONE', *, *, #3732, .F. ) ;
#20630=EDGE_CURVE ( 'NONE', #15727, #18296, #12058, .T. ) ;
#20633=VERTEX_POINT ( 'NONE', #4630 ) ;
#20659=PLANE ( 'NONE',  #6743 ) ;
#20678=ORIENTED_EDGE ( 'NONE', *, *, #19033, .F. ) ;
#20686=DIRECTION ( 'NONE',  ( 0.000000000000000000, -1.000000000000000000, 0.000000000000000000 ) ) ;
#20687=VECTOR ( 'NONE', #8609, 1000.000000000000000 ) ;
#20712=DIRECTION ( 'NONE',  ( 0.000000000000000000, -1.000000000000000000, 0.000000000000000000 ) ) ;
#20714=EDGE_LOOP ( 'NONE', ( #9446, #5403, #8604, #19736, #4418, #11861, #15878, #11214 ) ) ;
#20717=CARTESIAN_POINT ( 'NONE',  ( -47.83731665821552781, 10.00000000000000000, -38.93845529828707441 ) ) ;
#20740=( LENGTH_UNIT ( ) NAMED_UNIT ( * ) SI_UNIT ( .MILLI., .METRE. ) );
#20746=CARTESIAN_POINT ( 'NONE',  ( -35.00000000000000000, 22.00000000000000711, -14.99999999999997691 ) ) ;
#20757=VECTOR ( 'NONE', #21585, 1000.000000000000000 ) ;
#20763=AXIS2_PLACEMENT_3D ( 'NONE', #14398, #18195, #21755 ) ;
#20767=CARTESIAN_POINT ( 'NONE',  ( 35.00000000000000000, 10.00000000000000000, 41.00000000000002132 ) ) ;
#20770=DIRECTION ( 'NONE',  ( 0.000000000000000000, -1.000000000000000000, 0.000000000000000000 ) ) ;
#20791=ORIENTED_EDGE ( 'NONE', *, *, #21328, .T. ) ;
#20794=ORIENTED_EDGE ( 'NONE', *, *, #12957, .F. ) ;
#20796=CYLINDRICAL_SURFACE ( 'NONE', #179, 41.00000000000000000 ) ;
#20801=VECTOR ( 'NONE', #19449, 1000.000000000000114 ) ;
#20850=DIRECTION ( 'NONE',  ( 0.000000000000000000, -1.000000000000000000, 0.000000000000000000 ) ) ;
#20854=DIRECTION ( 'NONE',  ( 0.000000000000000000, -1.000000000000000000, 0.000000000000000000 ) ) ;
#20869=ORIENTED_EDGE ( 'NONE', *, *, #19445, .F. ) ;
#20884=CARTESIAN_POINT ( 'NONE',  ( 42.50000000000000000, 10.00000000000000000, 44.99999999999999289 ) ) ;
#20885=CIRCLE ( 'NONE', #14263, 2.500000000000002220 ) ;
#20891=ORIENTED_EDGE ( 'NONE', *, *, #748, .T. ) ;
#20892=DIRECTION ( 'NONE',  ( -1.067522139062650671E-15, 0.000000000000000000, -1.000000000000000000 ) ) ;
#20912=DIRECTION ( 'NONE',  ( 0.000000000000000000, -1.000000000000000000, 0.000000000000000000 ) ) ;
#20937=DIRECTION ( 'NONE',  ( 0.000000000000000000, -1.000000000000000000, 0.000000000000000000 ) ) ;
#20947=DIRECTION ( 'NONE',  ( 0.000000000000000000, -1.000000000000000000, 0.000000000000000000 ) ) ;
#20964=ORIENTED_EDGE ( 'NONE', *, *, #14597, .F. ) ;
#21007=ORIENTED_EDGE ( 'NONE', *, *, #6240, .T. ) ;
#21040=FACE_OUTER_BOUND ( 'NONE', #12214, .T. ) ;
#21054=DIRECTION ( 'NONE',  ( -0.000000000000000000, 1.000000000000000000, -0.000000000000000000 ) ) ;
#21055=CARTESIAN_POINT ( 'NONE',  ( 35.00000000000000000, 0.000000000000000000, 41.00000000000002132 ) ) ;
#21070=FACE_BOUND ( 'NONE', #242, .T. ) ;
#21104=VERTEX_POINT ( 'NONE', #18682 ) ;
#21129=CARTESIAN_POINT ( 'NONE',  ( -35.00000000000000000, 22.00000000000000355, -16.99999999999997868 ) ) ;
#21138=ADVANCED_BREP_SHAPE_REPRESENTATION ( '', ( #10617, #18273 ), #22313 ) ;
#21146=ORIENTED_EDGE ( 'NONE', *, *, #18187, .F. ) ;
#21149=PLANE ( 'NONE',  #1937 ) ;
#21159=CARTESIAN_POINT ( 'NONE',  ( 35.00000000000000000, 17.00000000000000000, 39.00000000000003553 ) ) ;
#21203=CARTESIAN_POINT ( 'NONE',  ( -42.49999999999996447, 10.00000000000000000, -45.00000000000000711 ) ) ;
#21220=LINE ( 'NONE', #8844, #10074 ) ;
#21223=CIRCLE ( 'NONE', #12427, 6.499999999999999112 ) ;
#21238=ORIENTED_EDGE ( 'NONE', *, *, #4426, .F. ) ;
#21253=EDGE_CURVE ( 'NONE', #18483, #15034, #12329, .T. ) ;
#21263=DIRECTION ( 'NONE',  ( -0.000000000000000000, -1.000000000000000000, -0.000000000000000000 ) ) ;
#21268=ORIENTED_EDGE ( 'NONE', *, *, #359, .T. ) ;
#21276=FACE_BOUND ( 'NONE', #3092, .T. ) ;
#21297=ORIENTED_EDGE ( 'NONE', *, *, #22489, .T. ) ;
#21305=DIRECTION ( 'NONE',  ( 0.000000000000000000, 1.000000000000000000, 0.000000000000000000 ) ) ;
#21316=ORIENTED_EDGE ( 'NONE', *, *, #1810, .F. ) ;
#21326=AXIS2_PLACEMENT_3D ( 'NONE', #11613, #6123, #15141 ) ;
#21328=EDGE_CURVE ( 'NONE', #16891, #15727, #12693, .T. ) ;
#21344=DIRECTION ( 'NONE',  ( 0.000000000000000000, -1.000000000000000000, 0.000000000000000000 ) ) ;
#21350=LINE ( 'NONE', #837, #18982 ) ;
#21351=ORIENTED_EDGE ( 'NONE', *, *, #7358, .T. ) ;
#21373=PLANE ( 'NONE',  #19120 ) ;
#21380=DIRECTION ( 'NONE',  ( 0.000000000000000000, 0.000000000000000000, -1.000000000000000000 ) ) ;
#21445=AXIS2_PLACEMENT_3D ( 'NONE', #883, #17026, #15301 ) ;
#21446=VECTOR ( 'NONE', #14608, 1000.000000000000000 ) ;
#21453=ORIENTED_EDGE ( 'NONE', *, *, #3623, .T. ) ;
#21472=CYLINDRICAL_SURFACE ( 'NONE', #3904, 15.00000000000000000 ) ;
#21499=CARTESIAN_POINT ( 'NONE',  ( 36.06598984771572702, 10.00000000000000000, -48.42385786802028491 ) ) ;
#21512=AXIS2_PLACEMENT_3D ( 'NONE', #3065, #10036, #15649 ) ;
#21513=AXIS2_PLACEMENT_3D ( 'NONE', #9371, #20141, #12895 ) ;
#21546=VECTOR ( 'NONE', #12473, 1000.000000000000000 ) ;
#21550=LINE ( 'NONE', #7104, #21546 ) ;
#21565=VERTEX_POINT ( 'NONE', #5154 ) ;
#21575=ORIENTED_EDGE ( 'NONE', *, *, #17655, .T. ) ;
#21585=DIRECTION ( 'NONE',  ( -0.000000000000000000, -1.000000000000000000, -0.000000000000000000 ) ) ;
#21586=DIRECTION ( 'NONE',  ( -1.000000000000000000, 0.000000000000000000, -0.000000000000000000 ) ) ;
#21595=ORIENTED_EDGE ( 'NONE', *, *, #6597, .T. ) ;
#21609=ORIENTED_EDGE ( 'NONE', *, *, #19179, .T. ) ;
#21614=CARTESIAN_POINT ( 'NONE',  ( -42.49999999999996447, 10.00000000000000000, -50.00000000000000711 ) ) ;
#21618=AXIS2_PLACEMENT_3D ( 'NONE', #2157, #424, #6981 ) ;
#21621=ADVANCED_FACE ( 'NONE', ( #1359 ), #15430, .T. ) ;
#21624=VERTEX_POINT ( 'NONE', #15204 ) ;
#21652=AXIS2_PLACEMENT_3D ( 'NONE', #7474, #9084, #19749 ) ;
#21688=ORIENTED_EDGE ( 'NONE', *, *, #13247, .T. ) ;
#21690=LINE ( 'NONE', #17910, #7581 ) ;
#21693=VECTOR ( 'NONE', #6576, 1000.000000000000000 ) ;
#21700=VERTEX_POINT ( 'NONE', #2156 ) ;
#21728=CIRCLE ( 'NONE', #9628, 6.499999999999999112 ) ;
#21755=DIRECTION ( 'NONE',  ( 0.000000000000000000, 0.000000000000000000, -1.000000000000000000 ) ) ;
#21767=EDGE_LOOP ( 'NONE', ( #3083, #8102, #246, #9224 ) ) ;
#21768=AXIS2_PLACEMENT_3D ( 'NONE', #183, #21054, #1698 ) ;
#21787=CYLINDRICAL_SURFACE ( 'NONE', #12210, 15.00000000000000000 ) ;
#21796=AXIS2_PLACEMENT_3D ( 'NONE', #1930, #17735, #2042 ) ;
#21814=ORIENTED_EDGE ( 'NONE', *, *, #3782, .T. ) ;
#21835=CIRCLE ( 'NONE', #6829, 39.00000000000001421 ) ;
#21842=VERTEX_POINT ( 'NONE', #13006 ) ;
#21868=CARTESIAN_POINT ( 'NONE',  ( -35.00000000000000000, 25.00000000000000000, 2.365113165210053967E-14 ) ) ;
#21872=ORIENTED_EDGE ( 'NONE', *, *, #21328, .F. ) ;
#21917=EDGE_CURVE ( 'NONE', #15452, #13636, #5781, .T. ) ;
#21936=ORIENTED_EDGE ( 'NONE', *, *, #14863, .T. ) ;
#21938=EDGE_CURVE ( 'NONE', #3991, #3967, #11756, .T. ) ;
#21939=DIRECTION ( 'NONE',  ( -0.000000000000000000, 1.000000000000000000, -0.000000000000000000 ) ) ;
#21941=VERTEX_POINT ( 'NONE', #15299 ) ;
#21942=DIRECTION ( 'NONE',  ( 0.000000000000000000, -1.000000000000000000, 0.000000000000000000 ) ) ;
#21974=ORIENTED_EDGE ( 'NONE', *, *, #9755, .T. ) ;
#21976=CIRCLE ( 'NONE', #14251, 2.500000000000002220 ) ;
#21982=VECTOR ( 'NONE', #22453, 1000.000000000000000 ) ;
#21985=LINE ( 'NONE', #20257, #17871 ) ;
#21987=CARTESIAN_POINT ( 'NONE',  ( 42.49999999999998579, 10.00000000000000000, -47.49999999999997868 ) ) ;
#22004=DIRECTION ( 'NONE',  ( -0.000000000000000000, 1.000000000000000000, -0.000000000000000000 ) ) ;
#22025=DIRECTION ( 'NONE',  ( 0.000000000000000000, -1.000000000000000000, 0.000000000000000000 ) ) ;
#22051=ORIENTED_EDGE ( 'NONE', *, *, #19922, .F. ) ;
#22064=DIRECTION ( 'NONE',  ( 0.000000000000000000, 0.000000000000000000, -1.000000000000000000 ) ) ;
#22067=LINE ( 'NONE', #21614, #7158 ) ;
#22084=CIRCLE ( 'NONE', #15096, 15.00000000000000000 ) ;
#22093=CARTESIAN_POINT ( 'NONE',  ( -42.49999999999996447, 10.00000000000000000, -47.50000000000000711 ) ) ;
#22107=EDGE_CURVE ( 'NONE', #3556, #5472, #1386, .T. ) ;
#22123=CARTESIAN_POINT ( 'NONE',  ( 35.00000000000000000, 7.000000000000000000, 2.365113165210053967E-14 ) ) ;
#22132=CONICAL_SURFACE ( 'NONE', #19209, 39.00000000000001421, 0.7853981633974447263 ) ;
#22144=CARTESIAN_POINT ( 'NONE',  ( -35.00000000000000000, 17.00000000000000000, 17.00000000000002487 ) ) ;
#22177=DIRECTION ( 'NONE',  ( 0.000000000000000000, -1.000000000000000000, 0.000000000000000000 ) ) ;
#22192=ORIENTED_EDGE ( 'NONE', *, *, #13017, .F. ) ;
#22195=EDGE_CURVE ( 'NONE', #20081, #1054, #7630, .T. ) ;
#22199=DIRECTION ( 'NONE',  ( -1.000000000000000000, 0.000000000000000000, 0.000000000000000000 ) ) ;
#22211=EDGE_CURVE ( 'NONE', #22660, #13179, #3744, .T. ) ;
#22229=LINE ( 'NONE', #15210, #21982 ) ;
#22252=EDGE_LOOP ( 'NONE', ( #14935, #20137, #8406, #3772 ) ) ;
#22256=DIRECTION ( 'NONE',  ( 0.000000000000000000, 0.000000000000000000, -1.000000000000000000 ) ) ;
#22275=AXIS2_PLACEMENT_3D ( 'NONE', #8301, #7848, #11623 ) ;
#22278=AXIS2_PLACEMENT_3D ( 'NONE', #4289, #16421, #5996 ) ;
#22295=CIRCLE ( 'NONE', #11658, 17.00000000000000000 ) ;
#22313=( GEOMETRIC_REPRESENTATION_CONTEXT ( 3 ) GLOBAL_UNCERTAINTY_ASSIGNED_CONTEXT ( ( #14917 ) ) GLOBAL_UNIT_ASSIGNED_CONTEXT ( ( #4491, #18459, #15004 ) ) REPRESENTATION_CONTEXT ( 'NONE', 'WORKASPACE' ) );
#22325=LINE ( 'NONE', #6609, #7540 ) ;
#22327=LINE ( 'NONE', #6611, #15666 ) ;
#22341=ORIENTED_EDGE ( 'NONE', *, *, #8745, .T. ) ;
#22414=ADVANCED_FACE ( 'NONE', ( #8720, #10084 ), #15579, .T. ) ;
#22424=DIRECTION ( 'NONE',  ( -0.1421319796954322034, 0.000000000000000000, 0.9898477157360405787 ) ) ;
#22445=AXIS2_PLACEMENT_3D ( 'NONE', #17760, #17986, #2066 ) ;
#22453=DIRECTION ( 'NONE',  ( 0.000000000000000000, -1.000000000000000000, 0.000000000000000000 ) ) ;
#22489=EDGE_CURVE ( 'NONE', #15378, #3909, #6662, .T. ) ;
#22514=CIRCLE ( 'NONE', #21768, 6.499999999999999112 ) ;
#22518=FACE_OUTER_BOUND ( 'NONE', #5603, .T. ) ;
#22534=CARTESIAN_POINT ( 'NONE',  ( -42.49999999999996447, 10.00000000000000000, -47.50000000000000711 ) ) ;
#22549=DIRECTION ( 'NONE',  ( 0.000000000000000000, -0.000000000000000000, -1.000000000000000000 ) ) ;
#22554=EDGE_CURVE ( 'NONE', #13097, #15034, #21550, .T. ) ;
#22564=FACE_BOUND ( 'NONE', #2471, .T. ) ;
#22568=ADVANCED_FACE ( 'NONE', ( #4031 ), #3908, .F. ) ;
#22589=LINE ( 'NONE', #17746, #6432 ) ;
#22604=EDGE_LOOP ( 'NONE', ( #1530, #6156, #8395, #2151, #7627 ) ) ;
#22624=AXIS2_PLACEMENT_3D ( 'NONE', #16171, #484, #7481 ) ;
#22629=EDGE_LOOP ( 'NONE', ( #4554, #21351 ) ) ;
#22630=ORIENTED_EDGE ( 'NONE', *, *, #14322, .T. ) ;
#22631=VERTEX_POINT ( 'NONE', #21203 ) ;
#22652=VECTOR ( 'NONE', #10699, 1000.000000000000000 ) ;
#22660=VERTEX_POINT ( 'NONE', #4863 ) ;
#22668=DIRECTION ( 'NONE',  ( 0.000000000000000000, -1.000000000000000000, 0.000000000000000000 ) ) ;
#22673=ORIENTED_EDGE ( 'NONE', *, *, #13247, .F. ) ;
#22687=VERTEX_POINT ( 'NONE', #4973 ) ;
#22742=COLOUR_RGB('Off White',0.89,0.88,0.83);
#22743=FILL_AREA_STYLE_COLOUR('',#22742);
#22744=FILL_AREA_STYLE('',(#22743));
#22745=SURFACE_STYLE_FILL_AREA(#22744);
#22746=SURFACE_SIDE_STYLE('',(#22745));
#22747=SURFACE_STYLE_USAGE(.BOTH.,#22746);
#22748=PRESENTATION_STYLE_ASSIGNMENT((#22747));
ENDSEC;
END-ISO-10303-21;
